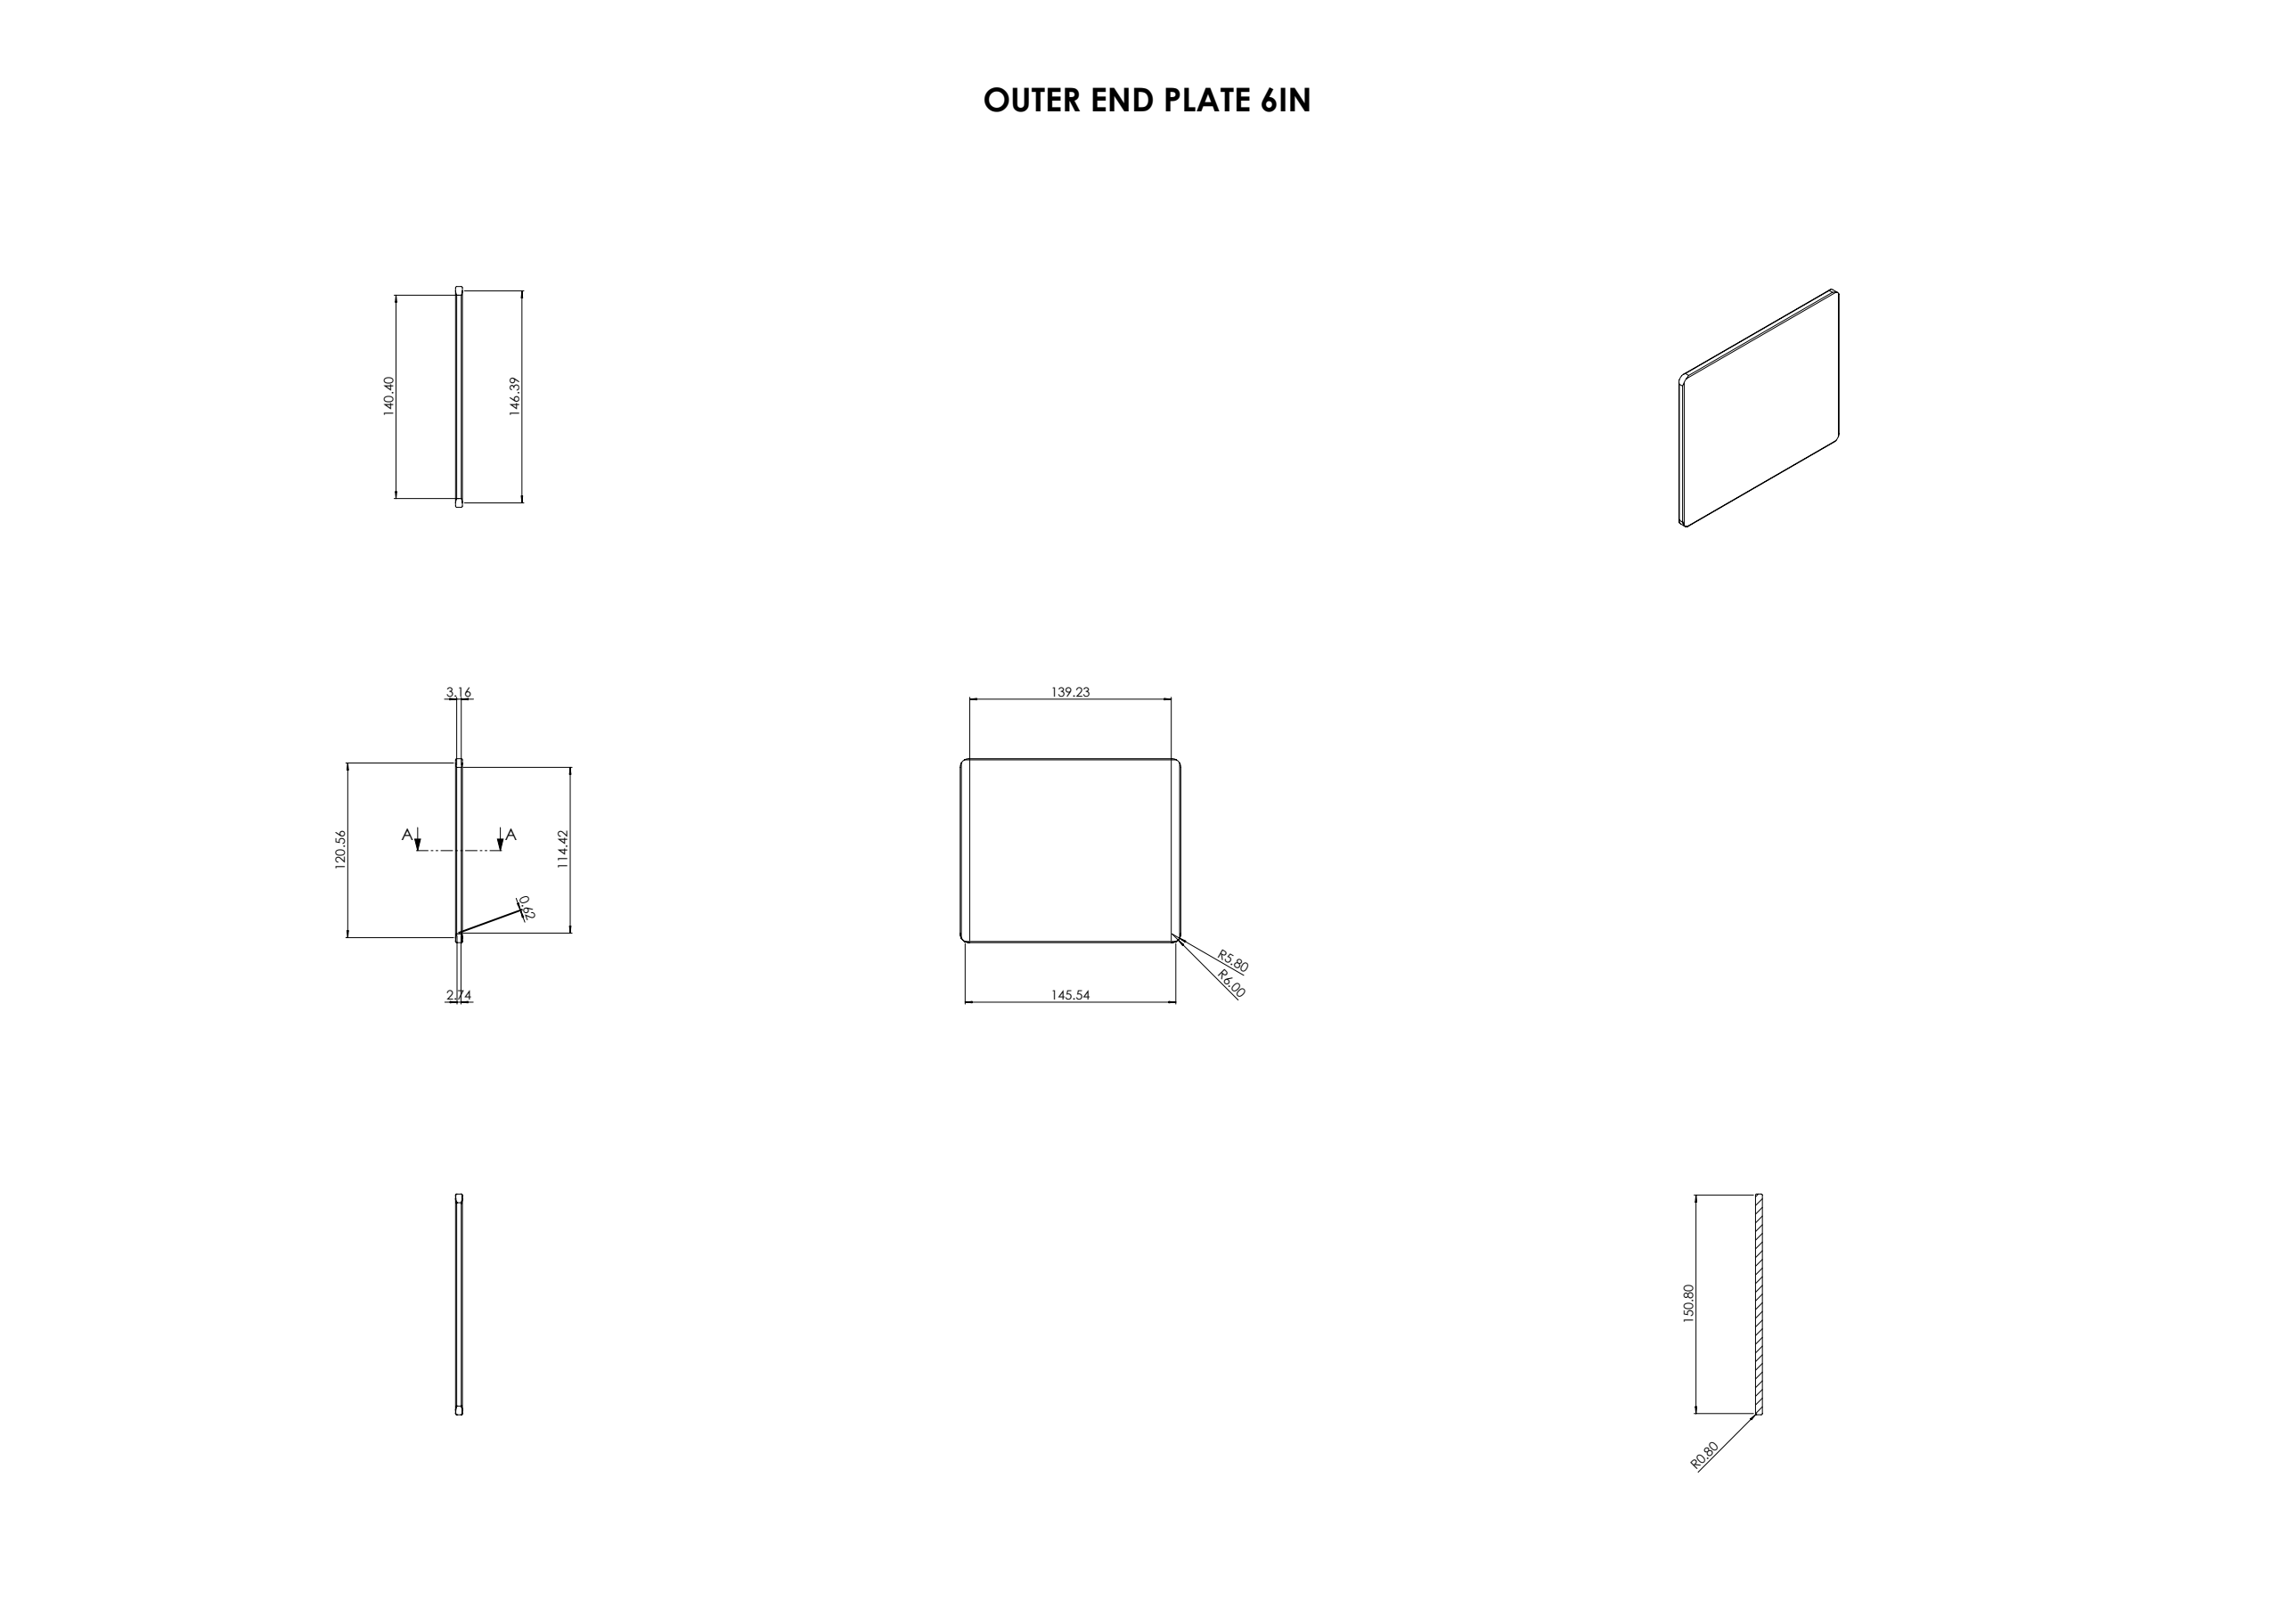
ISO-10303-21;
HEADER;
/* Generated by software containing ST-Developer
 * from STEP Tools, Inc. (www.steptools.com) 
 */

FILE_DESCRIPTION(
/* description */ (''),
/* implementation_level */ '2;1');

FILE_NAME(
/* name */ '02_Outer_End_Plate_6in.step',
/* time_stamp */ '2026-10-25T01:30:15-07:00',
/* author */ (''),
/* organization */ (''),
/* preprocessor_version */ 'ST-DEVELOPER v20.2',
/* originating_system */ 'Autodesk Translation Framework v15.15.0.0',
/* authorisation */ '');

FILE_SCHEMA (('AUTOMOTIVE_DESIGN { 1 0 10303 214 3 1 1 }'));
ENDSEC;

DATA;
#10=MECHANICAL_DESIGN_GEOMETRIC_PRESENTATION_REPRESENTATION('',(#564),#32309);
#88=B_SPLINE_CURVE_WITH_KNOTS('',3,(#18634,#18635,#18636,#18637,#18638,
#18639,#18640,#18641,#18642,#18643,#18644,#18645,#18646,#18647,#18648,#18649,
#18650,#18651,#18652,#18653,#18654,#18655,#18656,#18657,#18658,#18659,#18660,
#18661,#18662,#18663,#18664,#18665,#18666,#18667,#18668,#18669,#18670,#18671,
#18672,#18673,#18674,#18675,#18676,#18677,#18678,#18679,#18680,#18681,#18682,
#18683,#18684,#18685,#18686,#18687,#18688,#18689,#18690,#18691,#18692,#18693,
#18694,#18695,#18696,#18697,#18698,#18699,#18700,#18701,#18702,#18703,#18704,
#18705,#18706,#18707,#18708,#18709,#18710,#18711,#18712,#18713,#18714,#18715),
 .UNSPECIFIED.,.F.,.F.,(4,3,3,3,3,3,3,3,3,3,3,3,3,3,3,3,3,3,3,3,3,3,3,3,
3,3,3,4),(0.,0.0295705059520471,0.06051594873034,0.0926038163611335,0.126139587235275,
0.161619669140697,0.19997110729461,0.243460414926569,0.31097643988682,0.354040412393894,
0.394412886619275,0.429686040742309,0.462833625340497,0.494651029781358,
0.527129557828368,0.560643520110525,0.596019930687279,0.634095034705998,
0.676984118479283,0.757738088859462,0.799051739150417,0.836280907609681,
0.871099049046634,0.903485295335691,0.934889314251083,0.965468175632905,
0.995091329104342,1.),.UNSPECIFIED.);
#89=B_SPLINE_CURVE_WITH_KNOTS('',3,(#18717,#18718,#18719,#18720),
 .UNSPECIFIED.,.F.,.F.,(4,4),(-1.,0.),.UNSPECIFIED.);
#90=B_SPLINE_CURVE_WITH_KNOTS('',3,(#18722,#18723,#18724,#18725,#18726,
#18727,#18728,#18729,#18730,#18731,#18732,#18733,#18734,#18735,#18736,#18737,
#18738,#18739,#18740,#18741,#18742,#18743,#18744,#18745,#18746,#18747,#18748,
#18749,#18750,#18751,#18752,#18753,#18754,#18755,#18756,#18757,#18758,#18759,
#18760,#18761,#18762,#18763,#18764,#18765,#18766,#18767,#18768,#18769,#18770,
#18771,#18772,#18773),.UNSPECIFIED.,.F.,.F.,(4,3,3,3,3,3,3,3,3,3,3,3,3,
3,3,3,3,4),(0.,0.0499444618814776,0.102213228769125,0.161337745851018,0.226027786935006,
0.32277431356813,0.388018393772404,0.444871191794535,0.498045966144255,
0.551308035192963,0.608971249854249,0.676370629164652,0.757277971873489,
0.819640070739892,0.87628793152519,0.929442915859961,0.979183143018599,
1.),.UNSPECIFIED.);
#91=B_SPLINE_CURVE_WITH_KNOTS('',3,(#18813,#18814,#18815,#18816,#18817,
#18818,#18819,#18820,#18821,#18822,#18823,#18824,#18825,#18826,#18827,#18828,
#18829,#18830,#18831,#18832,#18833,#18834,#18835,#18836,#18837,#18838,#18839,
#18840,#18841,#18842,#18843,#18844,#18845,#18846,#18847,#18848,#18849,#18850,
#18851,#18852,#18853,#18854,#18855,#18856,#18857,#18858,#18859,#18860,#18861,
#18862,#18863,#18864),.UNSPECIFIED.,.F.,.F.,(4,3,3,3,3,3,3,3,3,3,3,3,3,
3,3,3,3,4),(0.,0.0499441833889704,0.102212663354794,0.161336814770105,0.226026300658832,
0.322773013076478,0.388016980146257,0.444869605985199,0.498043900535364,
0.551305760953485,0.608968431114082,0.676366602896629,0.757274952172472,
0.819637092644588,0.876284888158847,0.929439770312476,0.979179831895377,
1.),.UNSPECIFIED.);
#92=B_SPLINE_CURVE_WITH_KNOTS('',3,(#18866,#18867,#18868,#18869),
 .UNSPECIFIED.,.F.,.F.,(4,4),(0.,1.),.UNSPECIFIED.);
#93=B_SPLINE_CURVE_WITH_KNOTS('',3,(#18871,#18872,#18873,#18874,#18875,
#18876,#18877,#18878,#18879,#18880,#18881,#18882,#18883,#18884,#18885,#18886,
#18887,#18888,#18889,#18890,#18891,#18892,#18893,#18894,#18895,#18896,#18897,
#18898,#18899,#18900,#18901,#18902,#18903,#18904,#18905,#18906,#18907,#18908,
#18909,#18910,#18911,#18912,#18913,#18914,#18915,#18916,#18917,#18918,#18919,
#18920,#18921,#18922,#18923,#18924,#18925,#18926,#18927,#18928,#18929,#18930,
#18931,#18932,#18933,#18934,#18935,#18936,#18937,#18938,#18939,#18940,#18941,
#18942,#18943,#18944,#18945,#18946,#18947,#18948,#18949,#18950,#18951,#18952),
 .UNSPECIFIED.,.F.,.F.,(4,3,3,3,3,3,3,3,3,3,3,3,3,3,3,3,3,3,3,3,3,3,3,3,
3,3,3,4),(0.,0.0295773880527055,0.0605304168417959,0.0926266477934975,0.12617192252577,
0.16166335905183,0.200029751866471,0.243548698202303,0.31096188049889,0.354026762967709,
0.394400090282227,0.429679987033159,0.462839402284378,0.494661356434203,
0.527132671759088,0.560640873791091,0.596011156294116,0.634079510048534,
0.676959318035126,0.757719488526345,0.799022961860359,0.836244255344789,
0.871055470881663,0.903435211406727,0.934833076384915,0.965406058046024,
0.995023143022087,1.),.UNSPECIFIED.);
#94=B_SPLINE_CURVE_WITH_KNOTS('',3,(#18979,#18980,#18981,#18982,#18983,
#18984),.UNSPECIFIED.,.F.,.F.,(4,2,4),(9.99629094513137E-5,0.155241085196768,
0.273153287835105),.UNSPECIFIED.);
#95=B_SPLINE_CURVE_WITH_KNOTS('',3,(#18987,#18988,#18989,#18990,#18991,
#18992),.UNSPECIFIED.,.F.,.F.,(4,2,4),(-0.273153287835105,-0.155241085196768,
-9.99629094513137E-5),.UNSPECIFIED.);
#96=B_SPLINE_CURVE_WITH_KNOTS('',3,(#19018,#19019,#19020,#19021),
 .UNSPECIFIED.,.F.,.F.,(4,4),(-0.310482170393534,-0.273153287835093),
 .UNSPECIFIED.);
#97=B_SPLINE_CURVE_WITH_KNOTS('',3,(#19022,#19023,#19024,#19025),
 .UNSPECIFIED.,.F.,.F.,(4,4),(0.273153287835093,0.310482170393534),
 .UNSPECIFIED.);
#98=B_SPLINE_CURVE_WITH_KNOTS('',3,(#19051,#19052,#19053,#19054,#19055,
#19056),.UNSPECIFIED.,.F.,.F.,(4,2,4),(-0.954291288267864,-0.799150016166132,
-0.681237813527798),.UNSPECIFIED.);
#99=B_SPLINE_CURVE_WITH_KNOTS('',3,(#19059,#19060,#19061,#19062,#19063,
#19064),.UNSPECIFIED.,.F.,.F.,(4,2,4),(0.681237813527798,0.799150016166132,
0.954291288267864),.UNSPECIFIED.);
#100=B_SPLINE_CURVE_WITH_KNOTS('',3,(#19081,#19082,#19083,#19084),
 .UNSPECIFIED.,.F.,.F.,(4,4),(-0.681237813527811,-0.643908930969367),
 .UNSPECIFIED.);
#101=B_SPLINE_CURVE_WITH_KNOTS('',3,(#19085,#19086,#19087,#19088),
 .UNSPECIFIED.,.F.,.F.,(4,4),(0.643908930969367,0.681237813527811),
 .UNSPECIFIED.);
#102=B_SPLINE_CURVE_WITH_KNOTS('',3,(#19093,#19094,#19095,#19096,#19097,
#19098,#19099,#19100,#19101,#19102,#19103,#19104,#19105,#19106,#19107,#19108,
#19109,#19110,#19111,#19112,#19113,#19114,#19115,#19116,#19117,#19118,#19119,
#19120,#19121,#19122,#19123,#19124,#19125,#19126,#19127,#19128,#19129,#19130,
#19131,#19132,#19133,#19134,#19135,#19136,#19137,#19138,#19139,#19140,#19141,
#19142,#19143,#19144,#19145,#19146,#19147,#19148,#19149,#19150,#19151,#19152,
#19153,#19154,#19155,#19156,#19157,#19158,#19159,#19160,#19161,#19162,#19163,
#19164,#19165,#19166,#19167,#19168,#19169,#19170,#19171,#19172,#19173,#19174),
 .UNSPECIFIED.,.F.,.F.,(4,3,3,3,3,3,3,3,3,3,3,3,3,3,3,3,3,3,3,3,3,3,3,3,
3,3,3,4),(0.,0.0295773880962405,0.0605304169310475,0.0926266479315681,0.126171922717038,
0.161663359303526,0.200029752189728,0.243548698625291,0.310961878288235,
0.35402676089522,0.394400088339269,0.429679985266982,0.462839400402085,
0.494661354749945,0.527132670284999,0.560640872291038,0.596011154748267,
0.634079508418766,0.676959316170582,0.757719487127936,0.79902296069953,
0.836244254323238,0.871055469962877,0.903435210560169,0.9348330756024,0.965406057321837,
0.995023142345411,1.),.UNSPECIFIED.);
#103=B_SPLINE_CURVE_WITH_KNOTS('',3,(#19176,#19177,#19178,#19179,#19180,
#19181),.UNSPECIFIED.,.F.,.F.,(4,2,4),(-0.273153287835103,-0.155241085196768,
-9.99629094513097E-5),.UNSPECIFIED.);
#104=B_SPLINE_CURVE_WITH_KNOTS('',3,(#19199,#19200,#19201,#19202,#19203,
#19204,#19205,#19206,#19207,#19208,#19209,#19210,#19211,#19212,#19213,#19214,
#19215,#19216,#19217,#19218,#19219,#19220,#19221,#19222,#19223,#19224,#19225,
#19226,#19227,#19228,#19229,#19230,#19231,#19232,#19233,#19234,#19235,#19236,
#19237,#19238,#19239,#19240,#19241,#19242,#19243,#19244,#19245,#19246,#19247,
#19248,#19249,#19250),.UNSPECIFIED.,.F.,.F.,(4,3,3,3,3,3,3,3,3,3,3,3,3,
3,3,3,3,4),(0.,0.0499444622917576,0.102213229604467,0.161337747231124,0.226027789147348,
0.32277431550393,0.388018395851454,0.444871194115429,0.498045969164268,
0.551308038550752,0.608971254052268,0.676370635217512,0.757277976413134,
0.81964007522294,0.876287936115381,0.929442920613543,0.979183148031846,
1.),.UNSPECIFIED.);
#105=B_SPLINE_CURVE_WITH_KNOTS('',3,(#19252,#19253,#19254,#19255,#19256,
#19257),.UNSPECIFIED.,.F.,.F.,(4,2,4),(0.681229980645395,0.79914218328373,
0.954283455385462),.UNSPECIFIED.);
#106=B_SPLINE_CURVE_WITH_KNOTS('',3,(#19259,#19260,#19261,#19262),
 .UNSPECIFIED.,.F.,.F.,(4,4),(0.643901098086962,0.681229980645409),
 .UNSPECIFIED.);
#107=B_SPLINE_CURVE_WITH_KNOTS('',3,(#19266,#19267,#19268,#19269),
 .UNSPECIFIED.,.F.,.F.,(4,4),(0.269588855200382,0.305932679404608),
 .UNSPECIFIED.);
#108=B_SPLINE_CURVE_WITH_KNOTS('',3,(#19271,#19272,#19273,#19274,#19275,
#19276),.UNSPECIFIED.,.F.,.F.,(4,2,4),(9.97881403247492E-5,0.166940126137213,
0.269588855200419),.UNSPECIFIED.);
#109=B_SPLINE_CURVE_WITH_KNOTS('',3,(#19277,#19278,#19279,#19280,#19281,
#19282,#19283,#19284,#19285,#19286,#19287,#19288,#19289,#19290,#19291,#19292,
#19293,#19294,#19295,#19296,#19297,#19298,#19299,#19300,#19301,#19302,#19303,
#19304,#19305,#19306,#19307,#19308,#19309,#19310,#19311,#19312,#19313,#19314,
#19315,#19316,#19317,#19318,#19319,#19320,#19321,#19322,#19323,#19324,#19325,
#19326,#19327,#19328),.UNSPECIFIED.,.F.,.F.,(4,3,3,3,3,3,3,3,3,3,3,3,3,
3,3,3,3,4),(0.,0.0499444877726433,0.102213281220285,0.161337835137364,0.226027936148337,
0.322774444129795,0.38801851522186,0.444871319243691,0.498046130430203,
0.551308243614294,0.608971537556607,0.676371082027953,0.757278311520965,
0.819640416091138,0.876288295150041,0.92944330183216,0.979183558774527,
1.),.UNSPECIFIED.);
#110=B_SPLINE_CURVE_WITH_KNOTS('',3,(#19351,#19352,#19353,#19354,#19355,
#19356,#19357,#19358,#19359,#19360,#19361,#19362,#19363,#19364,#19365,#19366,
#19367,#19368,#19369,#19370,#19371,#19372,#19373,#19374,#19375,#19376,#19377,
#19378,#19379,#19380,#19381,#19382,#19383,#19384,#19385,#19386,#19387,#19388,
#19389,#19390,#19391,#19392,#19393,#19394,#19395,#19396,#19397,#19398,#19399,
#19400,#19401,#19402,#19403,#19404,#19405,#19406,#19407,#19408,#19409,#19410,
#19411,#19412,#19413,#19414,#19415,#19416,#19417,#19418,#19419,#19420,#19421,
#19422,#19423,#19424,#19425,#19426,#19427,#19428,#19429,#19430,#19431,#19432),
 .UNSPECIFIED.,.F.,.F.,(4,3,3,3,3,3,3,3,3,3,3,3,3,3,3,3,3,3,3,3,3,3,3,3,
3,3,3,4),(0.,0.0295705062457886,0.0605159494602176,0.0926038176850879,0.126139589401718,
0.161619672576972,0.199971112846056,0.243460425882021,0.310976395562794,
0.35404037084012,0.394412847662612,0.429686002557242,0.462833578893964,
0.494650986322964,0.527129524428408,0.560643490399518,0.596019903970715,
0.634095009431096,0.67698408832498,0.757738066243735,0.799051737694099,
0.836280920233922,0.87109907297074,0.903485328812536,0.934889356536429,
0.965468226164381,0.995091387717599,1.),.UNSPECIFIED.);
#111=B_SPLINE_CURVE_WITH_KNOTS('',3,(#19434,#19435,#19436,#19437),
 .UNSPECIFIED.,.F.,.F.,(4,4),(-1.,0.),.UNSPECIFIED.);
#112=B_SPLINE_CURVE_WITH_KNOTS('',3,(#19439,#19440,#19441,#19442,#19443,
#19444,#19445,#19446,#19447,#19448,#19449,#19450,#19451,#19452,#19453,#19454,
#19455,#19456,#19457,#19458,#19459,#19460,#19461,#19462,#19463,#19464,#19465,
#19466,#19467,#19468,#19469,#19470,#19471,#19472,#19473,#19474,#19475,#19476,
#19477,#19478,#19479,#19480,#19481,#19482,#19483,#19484,#19485,#19486,#19487,
#19488,#19489,#19490),.UNSPECIFIED.,.F.,.F.,(4,3,3,3,3,3,3,3,3,3,3,3,3,
3,3,3,3,4),(0.,0.049944493509105,0.102213293185184,0.161337852934914,0.226027959979003,
0.322774464981628,0.388018552338671,0.444871367106078,0.498046192643883,
0.551308282903018,0.608971555280469,0.676371064186631,0.757278298139973,
0.81964039022404,0.87628825630229,0.929443250152998,0.979183493767421,1.),
 .UNSPECIFIED.);
#113=B_SPLINE_CURVE_WITH_KNOTS('',3,(#19529,#19530,#19531,#19532,#19533,
#19534,#19535,#19536,#19537,#19538,#19539,#19540,#19541,#19542,#19543,#19544,
#19545,#19546,#19547,#19548,#19549,#19550,#19551,#19552,#19553,#19554,#19555,
#19556,#19557,#19558,#19559,#19560,#19561,#19562,#19563,#19564,#19565,#19566,
#19567,#19568,#19569,#19570,#19571,#19572,#19573,#19574,#19575,#19576,#19577,
#19578,#19579,#19580),.UNSPECIFIED.,.F.,.F.,(4,3,3,3,3,3,3,3,3,3,3,3,3,
3,3,3,3,4),(0.,0.0499441828918079,0.102212662342561,0.161336813097488,0.226026297979579,
0.322773010732132,0.388016977629376,0.444869603175185,0.498043896877559,
0.551305756885345,0.608968426026964,0.676366595561391,0.757274946671043,
0.819637087211295,0.876284882595595,0.929439764551152,0.979179825819233,
1.),.UNSPECIFIED.);
#114=B_SPLINE_CURVE_WITH_KNOTS('',3,(#19581,#19582,#19583,#19584),
 .UNSPECIFIED.,.F.,.F.,(4,4),(0.,1.),.UNSPECIFIED.);
#115=B_SPLINE_CURVE_WITH_KNOTS('',3,(#19610,#19611,#19612,#19613,#19614,
#19615),.UNSPECIFIED.,.F.,.F.,(4,2,4),(9.99629094513097E-5,0.155241085196768,
0.273153287835103),.UNSPECIFIED.);
#116=B_SPLINE_CURVE_WITH_KNOTS('',3,(#19642,#19643,#19644,#19645),
 .UNSPECIFIED.,.F.,.F.,(4,4),(-0.310482170393536,-0.273153287835089),
 .UNSPECIFIED.);
#117=B_SPLINE_CURVE_WITH_KNOTS('',3,(#19646,#19647,#19648,#19649),
 .UNSPECIFIED.,.F.,.F.,(4,4),(0.273153287835089,0.310482170393536),
 .UNSPECIFIED.);
#118=B_SPLINE_CURVE_WITH_KNOTS('',3,(#19675,#19676,#19677,#19678,#19679,
#19680),.UNSPECIFIED.,.F.,.F.,(4,2,4),(-0.945184496035906,-0.778344160365421,
-0.675695431302217),.UNSPECIFIED.);
#119=B_SPLINE_CURVE_WITH_KNOTS('',3,(#19683,#19684,#19685,#19686,#19687,
#19688),.UNSPECIFIED.,.F.,.F.,(4,2,4),(0.675695431302217,0.778344160365421,
0.945184496035906),.UNSPECIFIED.);
#120=B_SPLINE_CURVE_WITH_KNOTS('',3,(#19705,#19706,#19707,#19708),
 .UNSPECIFIED.,.F.,.F.,(4,4),(-0.675695431302254,-0.639351607098029),
 .UNSPECIFIED.);
#121=B_SPLINE_CURVE_WITH_KNOTS('',3,(#19709,#19710,#19711,#19712),
 .UNSPECIFIED.,.F.,.F.,(4,4),(0.639351607098029,0.675695431302254),
 .UNSPECIFIED.);
#122=B_SPLINE_CURVE_WITH_KNOTS('',3,(#19744,#19745,#19746,#19747,#19748,
#19749,#19750,#19751,#19752,#19753,#19754,#19755,#19756,#19757,#19758,#19759,
#19760,#19761,#19762,#19763,#19764,#19765,#19766,#19767,#19768,#19769,#19770,
#19771,#19772,#19773,#19774,#19775,#19776,#19777,#19778,#19779,#19780,#19781,
#19782,#19783,#19784,#19785,#19786,#19787,#19788,#19789,#19790,#19791,#19792,
#19793,#19794,#19795,#19796,#19797,#19798,#19799,#19800,#19801,#19802,#19803,
#19804,#19805,#19806,#19807,#19808,#19809,#19810,#19811,#19812,#19813,#19814,
#19815,#19816,#19817,#19818,#19819,#19820,#19821,#19822,#19823,#19824,#19825),
 .UNSPECIFIED.,.F.,.F.,(4,3,3,3,3,3,3,3,3,3,3,3,3,3,3,3,3,3,3,3,3,3,3,3,
3,3,3,4),(0.,0.0295705062009041,0.0605159493680217,0.0926038175409483,0.126139589200587,
0.161619672306982,0.199971112488613,0.243460425357206,0.310976394321422,
0.354040369676333,0.394412846571562,0.429686001479307,0.46283357764396,
0.49465098512599,0.527129523295935,0.560643489155532,0.596019902588203,
0.634095007862749,0.676984086399807,0.757738064799855,0.799051736386075,
0.836280918968163,0.871099071720543,0.903485327550832,0.934889355257872,
0.965468224868288,0.995091386390381,1.),.UNSPECIFIED.);
#123=B_SPLINE_CURVE_WITH_KNOTS('',3,(#19827,#19828,#19829,#19830),
 .UNSPECIFIED.,.F.,.F.,(4,4),(-1.,0.),.UNSPECIFIED.);
#124=B_SPLINE_CURVE_WITH_KNOTS('',3,(#19831,#19832,#19833,#19834,#19835,
#19836,#19837,#19838,#19839,#19840,#19841,#19842,#19843,#19844,#19845,#19846,
#19847,#19848,#19849,#19850,#19851,#19852,#19853,#19854,#19855,#19856,#19857,
#19858,#19859,#19860,#19861,#19862,#19863,#19864,#19865,#19866,#19867,#19868,
#19869,#19870,#19871,#19872,#19873,#19874,#19875,#19876,#19877,#19878,#19879,
#19880,#19881,#19882),.UNSPECIFIED.,.F.,.F.,(4,3,3,3,3,3,3,3,3,3,3,3,3,
3,3,3,3,4),(0.,0.0499444940857239,0.102213294358374,0.161337854873708,0.226027963088782,
0.322774467702684,0.388018555259764,0.444871370367514,0.498046196889068,
0.551308287624491,0.608971561184033,0.676371072696357,0.757278304522268,
0.819640396527144,0.87628826275593,0.92944325683678,0.979183500816116,1.),
 .UNSPECIFIED.);
#125=B_SPLINE_CURVE_WITH_KNOTS('',3,(#19921,#19922,#19923,#19924,#19925,
#19926,#19927,#19928,#19929,#19930,#19931,#19932,#19933,#19934,#19935,#19936,
#19937,#19938,#19939,#19940,#19941,#19942,#19943,#19944,#19945,#19946,#19947,
#19948,#19949,#19950,#19951,#19952,#19953,#19954,#19955,#19956,#19957,#19958,
#19959,#19960,#19961,#19962,#19963,#19964,#19965,#19966,#19967,#19968,#19969,
#19970,#19971,#19972),.UNSPECIFIED.,.F.,.F.,(4,3,3,3,3,3,3,3,3,3,3,3,3,
3,3,3,3,4),(0.,0.0499441826826897,0.102212661917196,0.161336812394391,0.22602629685116,
0.322773009744765,0.388016976569652,0.444869601991809,0.498043895337266,
0.551305755172809,0.608968423886568,0.676366592477159,0.757274944357869,
0.819637084926596,0.876284880256139,0.929439762127755,0.979179823263689,
1.),.UNSPECIFIED.);
#126=B_SPLINE_CURVE_WITH_KNOTS('',3,(#19974,#19975,#19976,#19977),
 .UNSPECIFIED.,.F.,.F.,(4,4),(0.,1.),.UNSPECIFIED.);
#127=B_SPLINE_CURVE_WITH_KNOTS('',3,(#19979,#19980,#19981,#19982,#19983,
#19984,#19985,#19986,#19987,#19988,#19989,#19990,#19991,#19992,#19993,#19994,
#19995,#19996,#19997,#19998,#19999,#20000,#20001,#20002,#20003,#20004,#20005,
#20006,#20007,#20008,#20009,#20010,#20011,#20012,#20013,#20014,#20015,#20016,
#20017,#20018,#20019,#20020,#20021,#20022,#20023,#20024,#20025,#20026,#20027,
#20028,#20029,#20030,#20031,#20032,#20033,#20034,#20035,#20036,#20037,#20038,
#20039,#20040,#20041,#20042,#20043,#20044,#20045,#20046,#20047,#20048,#20049,
#20050,#20051,#20052,#20053,#20054,#20055,#20056,#20057,#20058,#20059,#20060),
 .UNSPECIFIED.,.F.,.F.,(4,3,3,3,3,3,3,3,3,3,3,3,3,3,3,3,3,3,3,3,3,3,3,3,
3,3,3,4),(0.,0.0295773881143737,0.0605304169685423,0.0926266479893201,0.126171922797343,
0.161663359409954,0.200029752325282,0.243548698800364,0.310961877359763,
0.354026760024778,0.394400087523229,0.429679984526457,0.462839399613297,
0.494661354046568,0.527132669669348,0.560640871664874,0.596011154103228,
0.63407950774038,0.676959315395981,0.757719486546985,0.799022960216542,
0.836244253898911,0.871055469579005,0.90343521020651,0.934833075276548,
0.965406057021946,0.995023142066622,1.),.UNSPECIFIED.);
#128=B_SPLINE_CURVE_WITH_KNOTS('',3,(#20087,#20088,#20089,#20090,#20091,
#20092),.UNSPECIFIED.,.F.,.F.,(4,2,4),(9.99629094513175E-5,0.155241085196768,
0.273153287835103),.UNSPECIFIED.);
#129=B_SPLINE_CURVE_WITH_KNOTS('',3,(#20095,#20096,#20097,#20098,#20099,
#20100),.UNSPECIFIED.,.F.,.F.,(4,2,4),(-0.273153287835103,-0.155241085196768,
-9.99629094513175E-5),.UNSPECIFIED.);
#130=B_SPLINE_CURVE_WITH_KNOTS('',3,(#20126,#20127,#20128,#20129),
 .UNSPECIFIED.,.F.,.F.,(4,4),(-0.310482170393535,-0.273153287835089),
 .UNSPECIFIED.);
#131=B_SPLINE_CURVE_WITH_KNOTS('',3,(#20130,#20131,#20132,#20133),
 .UNSPECIFIED.,.F.,.F.,(4,4),(0.273153287835089,0.310482170393535),
 .UNSPECIFIED.);
#132=B_SPLINE_CURVE_WITH_KNOTS('',3,(#20159,#20160,#20161,#20162,#20163,
#20164),.UNSPECIFIED.,.F.,.F.,(4,2,4),(-0.945184496035905,-0.778344160365423,
-0.67569543130222),.UNSPECIFIED.);
#133=B_SPLINE_CURVE_WITH_KNOTS('',3,(#20167,#20168,#20169,#20170,#20171,
#20172),.UNSPECIFIED.,.F.,.F.,(4,2,4),(0.67569543130222,0.778344160365423,
0.945184496035905),.UNSPECIFIED.);
#134=B_SPLINE_CURVE_WITH_KNOTS('',3,(#20189,#20190,#20191,#20192),
 .UNSPECIFIED.,.F.,.F.,(4,4),(-0.675695431302257,-0.639351607098027),
 .UNSPECIFIED.);
#135=B_SPLINE_CURVE_WITH_KNOTS('',3,(#20193,#20194,#20195,#20196),
 .UNSPECIFIED.,.F.,.F.,(4,4),(0.639351607098027,0.675695431302257),
 .UNSPECIFIED.);
#136=B_SPLINE_CURVE_WITH_KNOTS('',3,(#20199,#20200,#20201,#20202,#20203,
#20204,#20205,#20206,#20207,#20208,#20209,#20210,#20211,#20212,#20213,#20214,
#20215,#20216,#20217,#20218,#20219,#20220,#20221,#20222,#20223,#20224,#20225,
#20226,#20227,#20228,#20229,#20230,#20231,#20232,#20233,#20234,#20235,#20236,
#20237,#20238,#20239,#20240,#20241,#20242,#20243,#20244,#20245,#20246,#20247,
#20248,#20249,#20250,#20251,#20252,#20253,#20254,#20255,#20256,#20257,#20258,
#20259,#20260,#20261,#20262,#20263,#20264,#20265,#20266,#20267,#20268,#20269,
#20270,#20271,#20272,#20273,#20274,#20275,#20276,#20277,#20278,#20279,#20280),
 .UNSPECIFIED.,.F.,.F.,(4,3,3,3,3,3,3,3,3,3,3,3,3,3,3,3,3,3,3,3,3,3,3,3,
3,3,3,4),(0.,0.0295774172384458,0.0605304778777659,0.0926267436200908,0.126172057442769,
0.161663540018093,0.200029992233166,0.243549050668545,0.310961698223174,
0.354026592084225,0.394399930078961,0.429679866520511,0.462839301683719,
0.494661290298148,0.527132633260964,0.560640855188699,0.596011159218635,
0.634079537198202,0.676959378678976,0.757719534009232,0.799023032825097,
0.836244348173232,0.871055583738876,0.90343534360451,0.934833227096761,
0.965406226610612,0.9950233300335,1.),.UNSPECIFIED.);
#137=B_SPLINE_CURVE_WITH_KNOTS('',3,(#20282,#20283,#20284,#20285,#20286,
#20287),.UNSPECIFIED.,.F.,.F.,(4,2,4),(-0.269588855200419,-0.166940126137213,
-9.97881403247492E-5),.UNSPECIFIED.);
#138=B_SPLINE_CURVE_WITH_KNOTS('',3,(#20313,#20314,#20315,#20316,#20317,
#20318,#20319,#20320,#20321,#20322,#20323,#20324,#20325,#20326,#20327,#20328,
#20329,#20330,#20331,#20332,#20333,#20334,#20335,#20336,#20337,#20338,#20339,
#20340,#20341,#20342,#20343,#20344,#20345,#20346,#20347,#20348,#20349,#20350,
#20351,#20352,#20353,#20354,#20355,#20356,#20357,#20358,#20359,#20360,#20361,
#20362,#20363,#20364,#20365,#20366,#20367,#20368,#20369,#20370,#20371,#20372,
#20373,#20374,#20375,#20376,#20377,#20378,#20379,#20380,#20381,#20382,#20383,
#20384,#20385,#20386,#20387,#20388,#20389,#20390,#20391,#20392,#20393,#20394),
 .UNSPECIFIED.,.F.,.F.,(4,3,3,3,3,3,3,3,3,3,3,3,3,3,3,3,3,3,3,3,3,3,3,3,
3,3,3,4),(0.,0.0295705059225161,0.060515948666961,0.0926038162606335,0.126139587093134,
0.161619668950802,0.199971107042965,0.243460414554639,0.310976439007705,
0.354040411569723,0.394412885846616,0.429686039982354,0.462833624458519,
0.494651028937031,0.527129557030648,0.560643519234301,0.596019929713648,
0.634095033602234,0.676984117122705,0.757738087842029,0.799051738229506,
0.836280906721543,0.871099048168231,0.903485294448113,0.934889313350476,
0.96546817471544,0.995091328163233,1.),.UNSPECIFIED.);
#139=B_SPLINE_CURVE_WITH_KNOTS('',3,(#20395,#20396,#20397,#20398),
 .UNSPECIFIED.,.F.,.F.,(4,4),(-1.,0.),.UNSPECIFIED.);
#140=B_SPLINE_CURVE_WITH_KNOTS('',3,(#20436,#20437,#20438,#20439),
 .UNSPECIFIED.,.F.,.F.,(4,4),(0.,1.),.UNSPECIFIED.);
#141=B_SPLINE_CURVE_WITH_KNOTS('',3,(#20487,#20488,#20489,#20490),
 .UNSPECIFIED.,.F.,.F.,(4,4),(-0.305932679404608,-0.269588855200382),
 .UNSPECIFIED.);
#142=B_SPLINE_CURVE_WITH_KNOTS('',3,(#20516,#20517,#20518,#20519,#20520,
#20521),.UNSPECIFIED.,.F.,.F.,(4,2,4),(-0.954283455385462,-0.79914218328373,
-0.681229980645395),.UNSPECIFIED.);
#143=B_SPLINE_CURVE_WITH_KNOTS('',3,(#20539,#20540,#20541,#20542),
 .UNSPECIFIED.,.F.,.F.,(4,4),(-0.681229980645409,-0.643901098086962),
 .UNSPECIFIED.);
#144=B_SPLINE_CURVE_WITH_KNOTS('',3,(#20556,#20557,#20558,#20559,#20560,
#20561),.UNSPECIFIED.,.F.,.F.,(4,2,4),(0.,0.155241085196768,0.310482170393537),
 .UNSPECIFIED.);
#145=B_SPLINE_CURVE_WITH_KNOTS('',3,(#20565,#20566,#20567,#20568,#20569,
#20570),.UNSPECIFIED.,.F.,.F.,(4,2,4),(0.643901098086962,0.79914218328373,
0.954383268480499),.UNSPECIFIED.);
#146=B_SPLINE_CURVE_WITH_KNOTS('',3,(#20572,#20573,#20574,#20575,#20576,
#20577),.UNSPECIFIED.,.F.,.F.,(4,2,4),(0.,0.15524108519677,0.31048217039354),
 .UNSPECIFIED.);
#147=B_SPLINE_CURVE_WITH_KNOTS('',3,(#20580,#20581,#20582,#20583,#20584,
#20585),.UNSPECIFIED.,.F.,.F.,(4,2,4),(0.643901098086964,0.799142183283734,
0.954383268480504),.UNSPECIFIED.);
#148=B_SPLINE_CURVE_WITH_KNOTS('',3,(#20591,#20592,#20593,#20594,#20595,
#20596),.UNSPECIFIED.,.F.,.F.,(4,2,4),(0.,0.155241085196768,0.310482170393535),
 .UNSPECIFIED.);
#149=B_SPLINE_CURVE_WITH_KNOTS('',3,(#20601,#20602,#20603,#20604,#20605,
#20606),.UNSPECIFIED.,.F.,.F.,(4,2,4),(0.643901098086961,0.799142183283728,
0.954383268480496),.UNSPECIFIED.);
#150=B_SPLINE_CURVE_WITH_KNOTS('',3,(#20608,#20609,#20610,#20611,#20612,
#20613),.UNSPECIFIED.,.F.,.F.,(4,2,4),(0.,0.166940126137215,0.305932679404607),
 .UNSPECIFIED.);
#151=B_SPLINE_CURVE_WITH_KNOTS('',3,(#20616,#20617,#20618,#20619,#20620,
#20621),.UNSPECIFIED.,.F.,.F.,(4,2,4),(0.643908930969365,0.799150016166133,
0.954391101362901),.UNSPECIFIED.);
#407=B_SPLINE_SURFACE_WITH_KNOTS('',3,3,((#18612,#18613,#18614,#18615,#18616),
(#18617,#18618,#18619,#18620,#18621),(#18622,#18623,#18624,#18625,#18626),
(#18627,#18628,#18629,#18630,#18631)),.UNSPECIFIED.,.F.,.F.,.F.,(4,4),(4,
1,4),(0.,1.),(0.,0.571428571428571,1.),.UNSPECIFIED.);
#408=B_SPLINE_SURFACE_WITH_KNOTS('',3,3,((#18775,#18776,#18777,#18778,#18779,
#18780,#18781,#18782,#18783),(#18784,#18785,#18786,#18787,#18788,#18789,
#18790,#18791,#18792),(#18793,#18794,#18795,#18796,#18797,#18798,#18799,
#18800,#18801),(#18802,#18803,#18804,#18805,#18806,#18807,#18808,#18809,
#18810)),.UNSPECIFIED.,.F.,.F.,.F.,(4,4),(4,1,1,1,1,1,4),(0.,1.),(0.,0.214285714285714,
0.357142857142857,0.571428571428571,0.785714285714286,0.857142857142857,
1.),.UNSPECIFIED.);
#409=B_SPLINE_SURFACE_WITH_KNOTS('',3,3,((#18954,#18955,#18956,#18957,#18958,
#18959),(#18960,#18961,#18962,#18963,#18964,#18965),(#18966,#18967,#18968,
#18969,#18970,#18971),(#18972,#18973,#18974,#18975,#18976,#18977)),
 .UNSPECIFIED.,.F.,.F.,.F.,(4,4),(4,2,4),(0.,1.),(9.99629094513137E-5,0.155241085196768,
0.273153287835105),.UNSPECIFIED.);
#410=B_SPLINE_SURFACE_WITH_KNOTS('',3,3,((#19002,#19003,#19004,#19005),
(#19006,#19007,#19008,#19009),(#19010,#19011,#19012,#19013),(#19014,#19015,
#19016,#19017)),.UNSPECIFIED.,.F.,.F.,.F.,(4,4),(4,4),(0.,1.),(0.273153287835093,
0.310482170393534),.UNSPECIFIED.);
#411=B_SPLINE_SURFACE_WITH_KNOTS('',3,3,((#19026,#19027,#19028,#19029,#19030,
#19031),(#19032,#19033,#19034,#19035,#19036,#19037),(#19038,#19039,#19040,
#19041,#19042,#19043),(#19044,#19045,#19046,#19047,#19048,#19049)),
 .UNSPECIFIED.,.F.,.F.,.F.,(4,4),(4,2,4),(0.,1.),(0.681237813527798,0.799150016166132,
0.954291288267864),.UNSPECIFIED.);
#412=B_SPLINE_SURFACE_WITH_KNOTS('',3,3,((#19065,#19066,#19067,#19068),
(#19069,#19070,#19071,#19072),(#19073,#19074,#19075,#19076),(#19077,#19078,
#19079,#19080)),.UNSPECIFIED.,.F.,.F.,.F.,(4,4),(4,4),(0.,1.),(0.643908930969367,
0.681237813527811),.UNSPECIFIED.);
#413=B_SPLINE_SURFACE_WITH_KNOTS('',3,3,((#19329,#19330,#19331,#19332,#19333),
(#19334,#19335,#19336,#19337,#19338),(#19339,#19340,#19341,#19342,#19343),
(#19344,#19345,#19346,#19347,#19348)),.UNSPECIFIED.,.F.,.F.,.F.,(4,4),(4,
1,4),(0.,1.),(0.,0.571428571428571,1.),.UNSPECIFIED.);
#414=B_SPLINE_SURFACE_WITH_KNOTS('',3,3,((#19492,#19493,#19494,#19495,#19496,
#19497,#19498,#19499,#19500),(#19501,#19502,#19503,#19504,#19505,#19506,
#19507,#19508,#19509),(#19510,#19511,#19512,#19513,#19514,#19515,#19516,
#19517,#19518),(#19519,#19520,#19521,#19522,#19523,#19524,#19525,#19526,
#19527)),.UNSPECIFIED.,.F.,.F.,.F.,(4,4),(4,1,1,1,1,1,4),(0.,1.),(0.,0.214285714285714,
0.357142857142857,0.571428571428571,0.785714285714286,0.857142857142857,
1.),.UNSPECIFIED.);
#415=B_SPLINE_SURFACE_WITH_KNOTS('',3,3,((#19585,#19586,#19587,#19588,#19589,
#19590),(#19591,#19592,#19593,#19594,#19595,#19596),(#19597,#19598,#19599,
#19600,#19601,#19602),(#19603,#19604,#19605,#19606,#19607,#19608)),
 .UNSPECIFIED.,.F.,.F.,.F.,(4,4),(4,2,4),(0.,1.),(9.99629094513097E-5,0.155241085196768,
0.273153287835103),.UNSPECIFIED.);
#416=B_SPLINE_SURFACE_WITH_KNOTS('',3,3,((#19626,#19627,#19628,#19629),
(#19630,#19631,#19632,#19633),(#19634,#19635,#19636,#19637),(#19638,#19639,
#19640,#19641)),.UNSPECIFIED.,.F.,.F.,.F.,(4,4),(4,4),(0.,1.),(0.273153287835089,
0.310482170393536),.UNSPECIFIED.);
#417=B_SPLINE_SURFACE_WITH_KNOTS('',3,3,((#19650,#19651,#19652,#19653,#19654,
#19655),(#19656,#19657,#19658,#19659,#19660,#19661),(#19662,#19663,#19664,
#19665,#19666,#19667),(#19668,#19669,#19670,#19671,#19672,#19673)),
 .UNSPECIFIED.,.F.,.F.,.F.,(4,4),(4,2,4),(0.,1.),(0.675695431302217,0.778344160365421,
0.945184496035906),.UNSPECIFIED.);
#418=B_SPLINE_SURFACE_WITH_KNOTS('',3,3,((#19689,#19690,#19691,#19692),
(#19693,#19694,#19695,#19696),(#19697,#19698,#19699,#19700),(#19701,#19702,
#19703,#19704)),.UNSPECIFIED.,.F.,.F.,.F.,(4,4),(4,4),(0.,1.),(0.639351607098029,
0.675695431302254),.UNSPECIFIED.);
#419=B_SPLINE_SURFACE_WITH_KNOTS('',3,3,((#19723,#19724,#19725,#19726,#19727),
(#19728,#19729,#19730,#19731,#19732),(#19733,#19734,#19735,#19736,#19737),
(#19738,#19739,#19740,#19741,#19742)),.UNSPECIFIED.,.F.,.F.,.F.,(4,4),(4,
1,4),(0.,1.),(0.,0.571428571428571,1.),.UNSPECIFIED.);
#420=B_SPLINE_SURFACE_WITH_KNOTS('',3,3,((#19883,#19884,#19885,#19886,#19887,
#19888,#19889,#19890,#19891),(#19892,#19893,#19894,#19895,#19896,#19897,
#19898,#19899,#19900),(#19901,#19902,#19903,#19904,#19905,#19906,#19907,
#19908,#19909),(#19910,#19911,#19912,#19913,#19914,#19915,#19916,#19917,
#19918)),.UNSPECIFIED.,.F.,.F.,.F.,(4,4),(4,1,1,1,1,1,4),(0.,1.),(0.,0.214285714285714,
0.357142857142857,0.571428571428571,0.785714285714286,0.857142857142857,
1.),.UNSPECIFIED.);
#421=B_SPLINE_SURFACE_WITH_KNOTS('',3,3,((#20062,#20063,#20064,#20065,#20066,
#20067),(#20068,#20069,#20070,#20071,#20072,#20073),(#20074,#20075,#20076,
#20077,#20078,#20079),(#20080,#20081,#20082,#20083,#20084,#20085)),
 .UNSPECIFIED.,.F.,.F.,.F.,(4,4),(4,2,4),(0.,1.),(9.99629094513175E-5,0.155241085196768,
0.273153287835103),.UNSPECIFIED.);
#422=B_SPLINE_SURFACE_WITH_KNOTS('',3,3,((#20110,#20111,#20112,#20113),
(#20114,#20115,#20116,#20117),(#20118,#20119,#20120,#20121),(#20122,#20123,
#20124,#20125)),.UNSPECIFIED.,.F.,.F.,.F.,(4,4),(4,4),(0.,1.),(0.273153287835089,
0.310482170393535),.UNSPECIFIED.);
#423=B_SPLINE_SURFACE_WITH_KNOTS('',3,3,((#20134,#20135,#20136,#20137,#20138,
#20139),(#20140,#20141,#20142,#20143,#20144,#20145),(#20146,#20147,#20148,
#20149,#20150,#20151),(#20152,#20153,#20154,#20155,#20156,#20157)),
 .UNSPECIFIED.,.F.,.F.,.F.,(4,4),(4,2,4),(0.,1.),(0.67569543130222,0.778344160365423,
0.945184496035905),.UNSPECIFIED.);
#424=B_SPLINE_SURFACE_WITH_KNOTS('',3,3,((#20173,#20174,#20175,#20176),
(#20177,#20178,#20179,#20180),(#20181,#20182,#20183,#20184),(#20185,#20186,
#20187,#20188)),.UNSPECIFIED.,.F.,.F.,.F.,(4,4),(4,4),(0.,1.),(0.639351607098027,
0.675695431302257),.UNSPECIFIED.);
#425=B_SPLINE_SURFACE_WITH_KNOTS('',3,3,((#20291,#20292,#20293,#20294,#20295),
(#20296,#20297,#20298,#20299,#20300),(#20301,#20302,#20303,#20304,#20305),
(#20306,#20307,#20308,#20309,#20310)),.UNSPECIFIED.,.F.,.F.,.F.,(4,4),(4,
1,4),(0.,1.),(0.,0.571428571428571,1.),.UNSPECIFIED.);
#426=B_SPLINE_SURFACE_WITH_KNOTS('',3,3,((#20400,#20401,#20402,#20403,#20404,
#20405,#20406,#20407,#20408),(#20409,#20410,#20411,#20412,#20413,#20414,
#20415,#20416,#20417),(#20418,#20419,#20420,#20421,#20422,#20423,#20424,
#20425,#20426),(#20427,#20428,#20429,#20430,#20431,#20432,#20433,#20434,
#20435)),.UNSPECIFIED.,.F.,.F.,.F.,(4,4),(4,1,1,1,1,1,4),(0.,1.),(0.,0.214285714285714,
0.357142857142857,0.571428571428571,0.785714285714286,0.857142857142857,
1.),.UNSPECIFIED.);
#427=B_SPLINE_SURFACE_WITH_KNOTS('',3,3,((#20440,#20441,#20442,#20443,#20444,
#20445),(#20446,#20447,#20448,#20449,#20450,#20451),(#20452,#20453,#20454,
#20455,#20456,#20457),(#20458,#20459,#20460,#20461,#20462,#20463)),
 .UNSPECIFIED.,.F.,.F.,.F.,(4,4),(4,2,4),(0.,1.),(9.97881403247492E-5,0.166940126137213,
0.269588855200419),.UNSPECIFIED.);
#428=B_SPLINE_SURFACE_WITH_KNOTS('',3,3,((#20471,#20472,#20473,#20474),
(#20475,#20476,#20477,#20478),(#20479,#20480,#20481,#20482),(#20483,#20484,
#20485,#20486)),.UNSPECIFIED.,.F.,.F.,.F.,(4,4),(4,4),(0.,1.),(0.269588855200382,
0.305932679404608),.UNSPECIFIED.);
#429=B_SPLINE_SURFACE_WITH_KNOTS('',3,3,((#20491,#20492,#20493,#20494,#20495,
#20496),(#20497,#20498,#20499,#20500,#20501,#20502),(#20503,#20504,#20505,
#20506,#20507,#20508),(#20509,#20510,#20511,#20512,#20513,#20514)),
 .UNSPECIFIED.,.F.,.F.,.F.,(4,4),(4,2,4),(0.,1.),(0.681229980645395,0.79914218328373,
0.954283455385462),.UNSPECIFIED.);
#430=B_SPLINE_SURFACE_WITH_KNOTS('',3,3,((#20523,#20524,#20525,#20526),
(#20527,#20528,#20529,#20530),(#20531,#20532,#20533,#20534),(#20535,#20536,
#20537,#20538)),.UNSPECIFIED.,.F.,.F.,.F.,(4,4),(4,4),(0.,1.),(0.643901098086962,
0.681229980645409),.UNSPECIFIED.);
#536=SHAPE_REPRESENTATION_RELATIONSHIP('SRR','None',#32363,#550);
#550=ADVANCED_BREP_SHAPE_REPRESENTATION('',(#578),#32296);
#564=STYLED_ITEM('',(#32516),#578);
#578=MANIFOLD_SOLID_BREP('Body1',#13805);
#656=CYLINDRICAL_SURFACE('',#14064,0.8);
#657=CYLINDRICAL_SURFACE('',#14066,6.00000000000001);
#658=CYLINDRICAL_SURFACE('',#14077,0.8);
#659=CYLINDRICAL_SURFACE('',#14078,6.00000000000001);
#660=CYLINDRICAL_SURFACE('',#14084,0.8);
#661=CYLINDRICAL_SURFACE('',#14085,6.);
#662=CYLINDRICAL_SURFACE('',#14087,0.8);
#663=CYLINDRICAL_SURFACE('',#14088,0.8);
#664=CYLINDRICAL_SURFACE('',#14089,5.99999999999998);
#665=CYLINDRICAL_SURFACE('',#14091,0.8);
#666=CYLINDRICAL_SURFACE('',#14092,0.8);
#667=CYLINDRICAL_SURFACE('',#14094,0.8);
#807=CIRCLE('',#14062,6.00000000000001);
#808=CIRCLE('',#14063,5.80000000000001);
#809=CIRCLE('',#14067,6.00000000000001);
#810=CIRCLE('',#14069,6.00000000000001);
#811=CIRCLE('',#14070,5.80000000000001);
#812=CIRCLE('',#14072,5.99999999999998);
#813=CIRCLE('',#14073,6.);
#814=CIRCLE('',#14075,5.80000000000001);
#815=CIRCLE('',#14076,6.00000000000001);
#816=CIRCLE('',#14080,5.80000000000001);
#817=CIRCLE('',#14082,6.);
#818=CIRCLE('',#14083,5.99999999999998);
#1113=CONICAL_SURFACE('',#14061,5.90000000000001,0.785398163397448);
#1114=CONICAL_SURFACE('',#14068,5.90000000000001,0.785398163397451);
#1115=CONICAL_SURFACE('',#14074,5.90000000000001,0.785398163397451);
#1116=CONICAL_SURFACE('',#14079,5.90000000000001,0.785398163397448);
#1293=FACE_OUTER_BOUND('',#2096,.T.);
#1294=FACE_OUTER_BOUND('',#2097,.T.);
#1295=FACE_OUTER_BOUND('',#2098,.T.);
#1296=FACE_OUTER_BOUND('',#2099,.T.);
#1297=FACE_OUTER_BOUND('',#2100,.T.);
#1298=FACE_OUTER_BOUND('',#2101,.T.);
#1299=FACE_OUTER_BOUND('',#2102,.T.);
#1300=FACE_OUTER_BOUND('',#2103,.T.);
#1301=FACE_OUTER_BOUND('',#2104,.T.);
#1302=FACE_OUTER_BOUND('',#2105,.T.);
#1303=FACE_OUTER_BOUND('',#2106,.T.);
#1304=FACE_OUTER_BOUND('',#2107,.T.);
#1305=FACE_OUTER_BOUND('',#2108,.T.);
#1306=FACE_OUTER_BOUND('',#2109,.T.);
#1307=FACE_OUTER_BOUND('',#2110,.T.);
#1308=FACE_OUTER_BOUND('',#2111,.T.);
#1309=FACE_OUTER_BOUND('',#2112,.T.);
#1310=FACE_OUTER_BOUND('',#2113,.T.);
#1311=FACE_OUTER_BOUND('',#2114,.T.);
#1312=FACE_OUTER_BOUND('',#2115,.T.);
#1313=FACE_OUTER_BOUND('',#2116,.T.);
#1314=FACE_OUTER_BOUND('',#2117,.T.);
#1315=FACE_OUTER_BOUND('',#2118,.T.);
#1316=FACE_OUTER_BOUND('',#2119,.T.);
#1317=FACE_OUTER_BOUND('',#2120,.T.);
#1318=FACE_OUTER_BOUND('',#2121,.T.);
#1319=FACE_OUTER_BOUND('',#2122,.T.);
#1320=FACE_OUTER_BOUND('',#2123,.T.);
#1321=FACE_OUTER_BOUND('',#2124,.T.);
#1322=FACE_OUTER_BOUND('',#2125,.T.);
#1323=FACE_OUTER_BOUND('',#2126,.T.);
#1324=FACE_OUTER_BOUND('',#2127,.T.);
#1325=FACE_OUTER_BOUND('',#2128,.T.);
#1326=FACE_OUTER_BOUND('',#2129,.T.);
#1327=FACE_OUTER_BOUND('',#2130,.T.);
#1328=FACE_OUTER_BOUND('',#2131,.T.);
#1329=FACE_OUTER_BOUND('',#2132,.T.);
#1330=FACE_OUTER_BOUND('',#2133,.T.);
#1331=FACE_OUTER_BOUND('',#2134,.T.);
#1332=FACE_OUTER_BOUND('',#2135,.T.);
#1333=FACE_OUTER_BOUND('',#2136,.T.);
#1334=FACE_OUTER_BOUND('',#2137,.T.);
#1335=FACE_OUTER_BOUND('',#2138,.T.);
#1336=FACE_OUTER_BOUND('',#2139,.T.);
#1337=FACE_OUTER_BOUND('',#2140,.T.);
#1338=FACE_OUTER_BOUND('',#2141,.T.);
#2096=EDGE_LOOP('',(#8909,#8910,#8911,#8912));
#2097=EDGE_LOOP('',(#8913,#8914,#8915,#8916));
#2098=EDGE_LOOP('',(#8917,#8918,#8919,#8920));
#2099=EDGE_LOOP('',(#8921,#8922,#8923,#8924));
#2100=EDGE_LOOP('',(#8925,#8926,#8927,#8928));
#2101=EDGE_LOOP('',(#8929,#8930,#8931,#8932));
#2102=EDGE_LOOP('',(#8933,#8934,#8935,#8936));
#2103=EDGE_LOOP('',(#8937,#8938,#8939,#8940,#8941,#8942));
#2104=EDGE_LOOP('',(#8943,#8944,#8945,#8946,#8947,#8948,#8949,#8950));
#2105=EDGE_LOOP('',(#8951,#8952,#8953,#8954,#8955,#8956,#8957,#8958,#8959,
#8960,#8961,#8962,#8963,#8964,#8965,#8966));
#2106=EDGE_LOOP('',(#8967,#8968,#8969,#8970));
#2107=EDGE_LOOP('',(#8971,#8972,#8973,#8974));
#2108=EDGE_LOOP('',(#8975,#8976,#8977,#8978));
#2109=EDGE_LOOP('',(#8979,#8980,#8981,#8982));
#2110=EDGE_LOOP('',(#8983,#8984,#8985,#8986));
#2111=EDGE_LOOP('',(#8987,#8988,#8989,#8990));
#2112=EDGE_LOOP('',(#8991,#8992,#8993,#8994));
#2113=EDGE_LOOP('',(#8995,#8996,#8997,#8998,#8999,#9000,#9001,#9002,#9003,
#9004,#9005,#9006));
#2114=EDGE_LOOP('',(#9007,#9008,#9009,#9010));
#2115=EDGE_LOOP('',(#9011,#9012,#9013,#9014));
#2116=EDGE_LOOP('',(#9015,#9016,#9017,#9018));
#2117=EDGE_LOOP('',(#9019,#9020,#9021,#9022));
#2118=EDGE_LOOP('',(#9023,#9024,#9025,#9026));
#2119=EDGE_LOOP('',(#9027,#9028,#9029,#9030));
#2120=EDGE_LOOP('',(#9031,#9032,#9033,#9034));
#2121=EDGE_LOOP('',(#9035,#9036,#9037,#9038,#9039,#9040));
#2122=EDGE_LOOP('',(#9041,#9042,#9043,#9044,#9045,#9046,#9047,#9048,#9049,
#9050,#9051,#9052,#9053,#9054,#9055,#9056));
#2123=EDGE_LOOP('',(#9057,#9058,#9059,#9060));
#2124=EDGE_LOOP('',(#9061,#9062,#9063,#9064));
#2125=EDGE_LOOP('',(#9065,#9066,#9067,#9068));
#2126=EDGE_LOOP('',(#9069,#9070,#9071,#9072));
#2127=EDGE_LOOP('',(#9073,#9074,#9075,#9076));
#2128=EDGE_LOOP('',(#9077,#9078,#9079,#9080));
#2129=EDGE_LOOP('',(#9081,#9082,#9083,#9084));
#2130=EDGE_LOOP('',(#9085,#9086,#9087,#9088,#9089,#9090,#9091,#9092,#9093,
#9094,#9095,#9096));
#2131=EDGE_LOOP('',(#9097,#9098,#9099,#9100,#9101));
#2132=EDGE_LOOP('',(#9102,#9103,#9104,#9105,#9106,#9107,#9108,#9109));
#2133=EDGE_LOOP('',(#9110,#9111,#9112,#9113,#9114,#9115));
#2134=EDGE_LOOP('',(#9116,#9117,#9118,#9119,#9120));
#2135=EDGE_LOOP('',(#9121,#9122,#9123,#9124));
#2136=EDGE_LOOP('',(#9125,#9126,#9127,#9128,#9129,#9130,#9131,#9132));
#2137=EDGE_LOOP('',(#9133,#9134,#9135,#9136));
#2138=EDGE_LOOP('',(#9137,#9138,#9139,#9140));
#2139=EDGE_LOOP('',(#9141,#9142,#9143,#9144,#9145));
#2140=EDGE_LOOP('',(#9146,#9147,#9148,#9149,#9150,#9151));
#2141=EDGE_LOOP('',(#9152,#9153,#9154,#9155,#9156));
#2977=LINE('',#18774,#4288);
#2978=LINE('',#18953,#4289);
#2979=LINE('',#18986,#4290);
#2980=LINE('',#18996,#4291);
#2981=LINE('',#19000,#4292);
#2982=LINE('',#19058,#4293);
#2983=LINE('',#19091,#4294);
#2984=LINE('',#19182,#4295);
#2985=LINE('',#19185,#4296);
#2986=LINE('',#19187,#4297);
#2987=LINE('',#19189,#4298);
#2988=LINE('',#19191,#4299);
#2989=LINE('',#19193,#4300);
#2990=LINE('',#19194,#4301);
#2991=LINE('',#19197,#4302);
#2992=LINE('',#19491,#4303);
#2993=LINE('',#19616,#4304);
#2994=LINE('',#19620,#4305);
#2995=LINE('',#19624,#4306);
#2996=LINE('',#19682,#4307);
#2997=LINE('',#19715,#4308);
#2998=LINE('',#19719,#4309);
#2999=LINE('',#19722,#4310);
#3000=LINE('',#20061,#4311);
#3001=LINE('',#20094,#4312);
#3002=LINE('',#20104,#4313);
#3003=LINE('',#20108,#4314);
#3004=LINE('',#20166,#4315);
#3005=LINE('',#20288,#4316);
#3006=LINE('',#20290,#4317);
#3007=LINE('',#20399,#4318);
#3008=LINE('',#20464,#4319);
#3009=LINE('',#20467,#4320);
#3010=LINE('',#20470,#4321);
#3011=LINE('',#20522,#4322);
#3012=LINE('',#20545,#4323);
#3013=LINE('',#20549,#4324);
#3014=LINE('',#20552,#4325);
#3015=LINE('',#20555,#4326);
#3016=LINE('',#20564,#4327);
#3017=LINE('',#20579,#4328);
#3018=LINE('',#20587,#4329);
#3019=LINE('',#20597,#4330);
#3020=LINE('',#20600,#4331);
#3021=LINE('',#20615,#4332);
#3022=LINE('',#20623,#4333);
#3023=LINE('',#20626,#4334);
#3024=LINE('',#20628,#4335);
#4288=VECTOR('',#15261,10.);
#4289=VECTOR('',#15262,10.);
#4290=VECTOR('',#15263,10.);
#4291=VECTOR('',#15266,10.);
#4292=VECTOR('',#15269,10.);
#4293=VECTOR('',#15272,10.);
#4294=VECTOR('',#15275,10.);
#4295=VECTOR('',#15276,10.);
#4296=VECTOR('',#15279,10.);
#4297=VECTOR('',#15280,10.);
#4298=VECTOR('',#15281,10.);
#4299=VECTOR('',#15282,10.);
#4300=VECTOR('',#15283,10.);
#4301=VECTOR('',#15284,10.);
#4302=VECTOR('',#15287,10.);
#4303=VECTOR('',#15290,10.);
#4304=VECTOR('',#15291,10.);
#4305=VECTOR('',#15294,10.);
#4306=VECTOR('',#15297,10.);
#4307=VECTOR('',#15300,10.);
#4308=VECTOR('',#15303,10.);
#4309=VECTOR('',#15306,10.);
#4310=VECTOR('',#15309,10.);
#4311=VECTOR('',#15310,10.);
#4312=VECTOR('',#15311,10.);
#4313=VECTOR('',#15314,10.);
#4314=VECTOR('',#15317,10.);
#4315=VECTOR('',#15320,10.);
#4316=VECTOR('',#15323,10.);
#4317=VECTOR('',#15326,10.);
#4318=VECTOR('',#15327,10.);
#4319=VECTOR('',#15328,10.);
#4320=VECTOR('',#15331,10.);
#4321=VECTOR('',#15334,10.);
#4322=VECTOR('',#15335,10.);
#4323=VECTOR('',#15338,10.);
#4324=VECTOR('',#15341,10.);
#4325=VECTOR('',#15344,10.);
#4326=VECTOR('',#15347,10.);
#4327=VECTOR('',#15350,10.);
#4328=VECTOR('',#15351,10.);
#4329=VECTOR('',#15354,10.);
#4330=VECTOR('',#15359,10.);
#4331=VECTOR('',#15362,10.);
#4332=VECTOR('',#15363,10.);
#4333=VECTOR('',#15366,10.);
#4334=VECTOR('',#15371,10.);
#4335=VECTOR('',#15374,10.);
#5584=VERTEX_POINT('',#18632);
#5585=VERTEX_POINT('',#18633);
#5586=VERTEX_POINT('',#18716);
#5587=VERTEX_POINT('',#18721);
#5588=VERTEX_POINT('',#18811);
#5589=VERTEX_POINT('',#18812);
#5590=VERTEX_POINT('',#18865);
#5591=VERTEX_POINT('',#18870);
#5592=VERTEX_POINT('',#18978);
#5593=VERTEX_POINT('',#18985);
#5594=VERTEX_POINT('',#18994);
#5595=VERTEX_POINT('',#18995);
#5596=VERTEX_POINT('',#18997);
#5597=VERTEX_POINT('',#18999);
#5598=VERTEX_POINT('',#19050);
#5599=VERTEX_POINT('',#19057);
#5600=VERTEX_POINT('',#19090);
#5601=VERTEX_POINT('',#19092);
#5602=VERTEX_POINT('',#19175);
#5603=VERTEX_POINT('',#19184);
#5604=VERTEX_POINT('',#19186);
#5605=VERTEX_POINT('',#19188);
#5606=VERTEX_POINT('',#19190);
#5607=VERTEX_POINT('',#19192);
#5608=VERTEX_POINT('',#19196);
#5609=VERTEX_POINT('',#19198);
#5610=VERTEX_POINT('',#19251);
#5611=VERTEX_POINT('',#19258);
#5612=VERTEX_POINT('',#19263);
#5613=VERTEX_POINT('',#19265);
#5614=VERTEX_POINT('',#19270);
#5615=VERTEX_POINT('',#19349);
#5616=VERTEX_POINT('',#19350);
#5617=VERTEX_POINT('',#19433);
#5618=VERTEX_POINT('',#19438);
#5619=VERTEX_POINT('',#19528);
#5620=VERTEX_POINT('',#19609);
#5621=VERTEX_POINT('',#19618);
#5622=VERTEX_POINT('',#19619);
#5623=VERTEX_POINT('',#19621);
#5624=VERTEX_POINT('',#19623);
#5625=VERTEX_POINT('',#19674);
#5626=VERTEX_POINT('',#19681);
#5627=VERTEX_POINT('',#19714);
#5628=VERTEX_POINT('',#19716);
#5629=VERTEX_POINT('',#19718);
#5630=VERTEX_POINT('',#19720);
#5631=VERTEX_POINT('',#19743);
#5632=VERTEX_POINT('',#19826);
#5633=VERTEX_POINT('',#19919);
#5634=VERTEX_POINT('',#19920);
#5635=VERTEX_POINT('',#19973);
#5636=VERTEX_POINT('',#19978);
#5637=VERTEX_POINT('',#20086);
#5638=VERTEX_POINT('',#20093);
#5639=VERTEX_POINT('',#20102);
#5640=VERTEX_POINT('',#20103);
#5641=VERTEX_POINT('',#20105);
#5642=VERTEX_POINT('',#20107);
#5643=VERTEX_POINT('',#20158);
#5644=VERTEX_POINT('',#20165);
#5645=VERTEX_POINT('',#20198);
#5646=VERTEX_POINT('',#20281);
#5647=VERTEX_POINT('',#20311);
#5648=VERTEX_POINT('',#20312);
#5649=VERTEX_POINT('',#20466);
#5650=VERTEX_POINT('',#20468);
#5651=VERTEX_POINT('',#20515);
#5652=VERTEX_POINT('',#20544);
#5653=VERTEX_POINT('',#20546);
#5654=VERTEX_POINT('',#20548);
#5655=VERTEX_POINT('',#20550);
#5656=VERTEX_POINT('',#20554);
#5657=VERTEX_POINT('',#20563);
#5658=VERTEX_POINT('',#20571);
#5659=VERTEX_POINT('',#20578);
#5660=VERTEX_POINT('',#20590);
#5661=VERTEX_POINT('',#20599);
#5662=VERTEX_POINT('',#20607);
#5663=VERTEX_POINT('',#20614);
#6831=EDGE_CURVE('',#5584,#5585,#88,.T.);
#6832=EDGE_CURVE('',#5586,#5585,#89,.T.);
#6833=EDGE_CURVE('',#5586,#5587,#90,.T.);
#6834=EDGE_CURVE('',#5587,#5584,#2977,.T.);
#6835=EDGE_CURVE('',#5588,#5589,#91,.T.);
#6836=EDGE_CURVE('',#5590,#5589,#92,.T.);
#6837=EDGE_CURVE('',#5590,#5591,#93,.T.);
#6838=EDGE_CURVE('',#5591,#5588,#2978,.T.);
#6839=EDGE_CURVE('',#5589,#5592,#94,.T.);
#6840=EDGE_CURVE('',#5592,#5593,#2979,.T.);
#6841=EDGE_CURVE('',#5593,#5590,#95,.T.);
#6842=EDGE_CURVE('',#5594,#5595,#2980,.T.);
#6843=EDGE_CURVE('',#5595,#5596,#807,.T.);
#6844=EDGE_CURVE('',#5596,#5597,#2981,.T.);
#6845=EDGE_CURVE('',#5597,#5594,#808,.T.);
#6846=EDGE_CURVE('',#5594,#5593,#96,.T.);
#6847=EDGE_CURVE('',#5592,#5595,#97,.T.);
#6848=EDGE_CURVE('',#5585,#5598,#98,.T.);
#6849=EDGE_CURVE('',#5598,#5599,#2982,.T.);
#6850=EDGE_CURVE('',#5599,#5586,#99,.T.);
#6851=EDGE_CURVE('',#5598,#5597,#100,.T.);
#6852=EDGE_CURVE('',#5596,#5599,#101,.T.);
#6853=EDGE_CURVE('',#5584,#5600,#2983,.T.);
#6854=EDGE_CURVE('',#5601,#5600,#102,.T.);
#6855=EDGE_CURVE('',#5602,#5601,#103,.T.);
#6856=EDGE_CURVE('',#5602,#5598,#2984,.T.);
#6857=EDGE_CURVE('',#5587,#5603,#2985,.T.);
#6858=EDGE_CURVE('',#5604,#5603,#2986,.T.);
#6859=EDGE_CURVE('',#5605,#5604,#2987,.T.);
#6860=EDGE_CURVE('',#5606,#5605,#2988,.T.);
#6861=EDGE_CURVE('',#5607,#5606,#2989,.T.);
#6862=EDGE_CURVE('',#5600,#5607,#2990,.T.);
#6863=EDGE_CURVE('',#5588,#5608,#2991,.T.);
#6864=EDGE_CURVE('',#5609,#5608,#104,.T.);
#6865=EDGE_CURVE('',#5610,#5609,#105,.T.);
#6866=EDGE_CURVE('',#5611,#5610,#106,.T.);
#6867=EDGE_CURVE('',#5612,#5611,#809,.T.);
#6868=EDGE_CURVE('',#5613,#5612,#107,.T.);
#6869=EDGE_CURVE('',#5614,#5613,#108,.T.);
#6870=EDGE_CURVE('',#5603,#5614,#109,.T.);
#6871=EDGE_CURVE('',#5615,#5616,#110,.T.);
#6872=EDGE_CURVE('',#5617,#5616,#111,.T.);
#6873=EDGE_CURVE('',#5617,#5618,#112,.T.);
#6874=EDGE_CURVE('',#5618,#5615,#2992,.T.);
#6875=EDGE_CURVE('',#5607,#5619,#113,.T.);
#6876=EDGE_CURVE('',#5601,#5619,#114,.T.);
#6877=EDGE_CURVE('',#5619,#5620,#115,.T.);
#6878=EDGE_CURVE('',#5620,#5602,#2993,.T.);
#6879=EDGE_CURVE('',#5621,#5622,#2994,.T.);
#6880=EDGE_CURVE('',#5622,#5623,#810,.T.);
#6881=EDGE_CURVE('',#5623,#5624,#2995,.T.);
#6882=EDGE_CURVE('',#5624,#5621,#811,.T.);
#6883=EDGE_CURVE('',#5621,#5602,#116,.T.);
#6884=EDGE_CURVE('',#5620,#5622,#117,.T.);
#6885=EDGE_CURVE('',#5616,#5625,#118,.T.);
#6886=EDGE_CURVE('',#5625,#5626,#2996,.T.);
#6887=EDGE_CURVE('',#5626,#5617,#119,.T.);
#6888=EDGE_CURVE('',#5625,#5624,#120,.T.);
#6889=EDGE_CURVE('',#5623,#5626,#121,.T.);
#6890=EDGE_CURVE('',#5627,#5625,#2997,.T.);
#6891=EDGE_CURVE('',#5628,#5627,#812,.T.);
#6892=EDGE_CURVE('',#5629,#5628,#2998,.T.);
#6893=EDGE_CURVE('',#5630,#5629,#813,.T.);
#6894=EDGE_CURVE('',#5593,#5630,#2999,.T.);
#6895=EDGE_CURVE('',#5605,#5631,#122,.T.);
#6896=EDGE_CURVE('',#5632,#5631,#123,.T.);
#6897=EDGE_CURVE('',#5632,#5606,#124,.T.);
#6898=EDGE_CURVE('',#5633,#5634,#125,.T.);
#6899=EDGE_CURVE('',#5635,#5634,#126,.T.);
#6900=EDGE_CURVE('',#5635,#5636,#127,.T.);
#6901=EDGE_CURVE('',#5636,#5633,#3000,.T.);
#6902=EDGE_CURVE('',#5634,#5637,#128,.T.);
#6903=EDGE_CURVE('',#5637,#5638,#3001,.T.);
#6904=EDGE_CURVE('',#5638,#5635,#129,.T.);
#6905=EDGE_CURVE('',#5639,#5640,#3002,.T.);
#6906=EDGE_CURVE('',#5640,#5641,#814,.T.);
#6907=EDGE_CURVE('',#5641,#5642,#3003,.T.);
#6908=EDGE_CURVE('',#5642,#5639,#815,.T.);
#6909=EDGE_CURVE('',#5641,#5638,#130,.T.);
#6910=EDGE_CURVE('',#5637,#5642,#131,.T.);
#6911=EDGE_CURVE('',#5631,#5643,#132,.T.);
#6912=EDGE_CURVE('',#5643,#5644,#3004,.T.);
#6913=EDGE_CURVE('',#5644,#5632,#133,.T.);
#6914=EDGE_CURVE('',#5643,#5640,#134,.T.);
#6915=EDGE_CURVE('',#5639,#5644,#135,.T.);
#6916=EDGE_CURVE('',#5645,#5604,#136,.T.);
#6917=EDGE_CURVE('',#5646,#5645,#137,.T.);
#6918=EDGE_CURVE('',#5646,#5643,#3005,.T.);
#6919=EDGE_CURVE('',#5618,#5633,#3006,.T.);
#6920=EDGE_CURVE('',#5647,#5648,#138,.T.);
#6921=EDGE_CURVE('',#5609,#5648,#139,.T.);
#6922=EDGE_CURVE('',#5608,#5647,#3007,.T.);
#6923=EDGE_CURVE('',#5645,#5614,#140,.T.);
#6924=EDGE_CURVE('',#5613,#5646,#3008,.T.);
#6925=EDGE_CURVE('',#5611,#5649,#3009,.T.);
#6926=EDGE_CURVE('',#5649,#5650,#816,.T.);
#6927=EDGE_CURVE('',#5650,#5612,#3010,.T.);
#6928=EDGE_CURVE('',#5650,#5646,#141,.T.);
#6929=EDGE_CURVE('',#5648,#5651,#142,.T.);
#6930=EDGE_CURVE('',#5651,#5610,#3011,.T.);
#6931=EDGE_CURVE('',#5651,#5649,#143,.T.);
#6932=EDGE_CURVE('',#5652,#5651,#3012,.T.);
#6933=EDGE_CURVE('',#5652,#5653,#817,.T.);
#6934=EDGE_CURVE('',#5654,#5653,#3013,.T.);
#6935=EDGE_CURVE('',#5654,#5655,#818,.T.);
#6936=EDGE_CURVE('',#5638,#5655,#3014,.T.);
#6937=EDGE_CURVE('',#5647,#5656,#3015,.T.);
#6938=EDGE_CURVE('',#5656,#5652,#144,.T.);
#6939=EDGE_CURVE('',#5657,#5656,#3016,.T.);
#6940=EDGE_CURVE('',#5630,#5657,#145,.T.);
#6941=EDGE_CURVE('',#5658,#5629,#146,.T.);
#6942=EDGE_CURVE('',#5658,#5659,#3017,.T.);
#6943=EDGE_CURVE('',#5653,#5659,#147,.T.);
#6944=EDGE_CURVE('',#5657,#5591,#3018,.T.);
#6945=EDGE_CURVE('',#5660,#5654,#148,.T.);
#6946=EDGE_CURVE('',#5659,#5660,#3019,.T.);
#6947=EDGE_CURVE('',#5661,#5660,#3020,.T.);
#6948=EDGE_CURVE('',#5628,#5661,#149,.T.);
#6949=EDGE_CURVE('',#5662,#5627,#150,.T.);
#6950=EDGE_CURVE('',#5662,#5663,#3021,.T.);
#6951=EDGE_CURVE('',#5655,#5663,#151,.T.);
#6952=EDGE_CURVE('',#5661,#5658,#3022,.T.);
#6953=EDGE_CURVE('',#5663,#5636,#3023,.T.);
#6954=EDGE_CURVE('',#5615,#5662,#3024,.T.);
#8909=ORIENTED_EDGE('',*,*,#6831,.T.);
#8910=ORIENTED_EDGE('',*,*,#6832,.F.);
#8911=ORIENTED_EDGE('',*,*,#6833,.T.);
#8912=ORIENTED_EDGE('',*,*,#6834,.T.);
#8913=ORIENTED_EDGE('',*,*,#6835,.T.);
#8914=ORIENTED_EDGE('',*,*,#6836,.F.);
#8915=ORIENTED_EDGE('',*,*,#6837,.T.);
#8916=ORIENTED_EDGE('',*,*,#6838,.T.);
#8917=ORIENTED_EDGE('',*,*,#6836,.T.);
#8918=ORIENTED_EDGE('',*,*,#6839,.T.);
#8919=ORIENTED_EDGE('',*,*,#6840,.T.);
#8920=ORIENTED_EDGE('',*,*,#6841,.T.);
#8921=ORIENTED_EDGE('',*,*,#6842,.T.);
#8922=ORIENTED_EDGE('',*,*,#6843,.T.);
#8923=ORIENTED_EDGE('',*,*,#6844,.T.);
#8924=ORIENTED_EDGE('',*,*,#6845,.T.);
#8925=ORIENTED_EDGE('',*,*,#6842,.F.);
#8926=ORIENTED_EDGE('',*,*,#6846,.T.);
#8927=ORIENTED_EDGE('',*,*,#6840,.F.);
#8928=ORIENTED_EDGE('',*,*,#6847,.T.);
#8929=ORIENTED_EDGE('',*,*,#6832,.T.);
#8930=ORIENTED_EDGE('',*,*,#6848,.T.);
#8931=ORIENTED_EDGE('',*,*,#6849,.T.);
#8932=ORIENTED_EDGE('',*,*,#6850,.T.);
#8933=ORIENTED_EDGE('',*,*,#6849,.F.);
#8934=ORIENTED_EDGE('',*,*,#6851,.T.);
#8935=ORIENTED_EDGE('',*,*,#6844,.F.);
#8936=ORIENTED_EDGE('',*,*,#6852,.T.);
#8937=ORIENTED_EDGE('',*,*,#6848,.F.);
#8938=ORIENTED_EDGE('',*,*,#6831,.F.);
#8939=ORIENTED_EDGE('',*,*,#6853,.T.);
#8940=ORIENTED_EDGE('',*,*,#6854,.F.);
#8941=ORIENTED_EDGE('',*,*,#6855,.F.);
#8942=ORIENTED_EDGE('',*,*,#6856,.T.);
#8943=ORIENTED_EDGE('',*,*,#6834,.F.);
#8944=ORIENTED_EDGE('',*,*,#6857,.T.);
#8945=ORIENTED_EDGE('',*,*,#6858,.F.);
#8946=ORIENTED_EDGE('',*,*,#6859,.F.);
#8947=ORIENTED_EDGE('',*,*,#6860,.F.);
#8948=ORIENTED_EDGE('',*,*,#6861,.F.);
#8949=ORIENTED_EDGE('',*,*,#6862,.F.);
#8950=ORIENTED_EDGE('',*,*,#6853,.F.);
#8951=ORIENTED_EDGE('',*,*,#6833,.F.);
#8952=ORIENTED_EDGE('',*,*,#6850,.F.);
#8953=ORIENTED_EDGE('',*,*,#6852,.F.);
#8954=ORIENTED_EDGE('',*,*,#6843,.F.);
#8955=ORIENTED_EDGE('',*,*,#6847,.F.);
#8956=ORIENTED_EDGE('',*,*,#6839,.F.);
#8957=ORIENTED_EDGE('',*,*,#6835,.F.);
#8958=ORIENTED_EDGE('',*,*,#6863,.T.);
#8959=ORIENTED_EDGE('',*,*,#6864,.F.);
#8960=ORIENTED_EDGE('',*,*,#6865,.F.);
#8961=ORIENTED_EDGE('',*,*,#6866,.F.);
#8962=ORIENTED_EDGE('',*,*,#6867,.F.);
#8963=ORIENTED_EDGE('',*,*,#6868,.F.);
#8964=ORIENTED_EDGE('',*,*,#6869,.F.);
#8965=ORIENTED_EDGE('',*,*,#6870,.F.);
#8966=ORIENTED_EDGE('',*,*,#6857,.F.);
#8967=ORIENTED_EDGE('',*,*,#6871,.T.);
#8968=ORIENTED_EDGE('',*,*,#6872,.F.);
#8969=ORIENTED_EDGE('',*,*,#6873,.T.);
#8970=ORIENTED_EDGE('',*,*,#6874,.T.);
#8971=ORIENTED_EDGE('',*,*,#6875,.T.);
#8972=ORIENTED_EDGE('',*,*,#6876,.F.);
#8973=ORIENTED_EDGE('',*,*,#6854,.T.);
#8974=ORIENTED_EDGE('',*,*,#6862,.T.);
#8975=ORIENTED_EDGE('',*,*,#6876,.T.);
#8976=ORIENTED_EDGE('',*,*,#6877,.T.);
#8977=ORIENTED_EDGE('',*,*,#6878,.T.);
#8978=ORIENTED_EDGE('',*,*,#6855,.T.);
#8979=ORIENTED_EDGE('',*,*,#6879,.T.);
#8980=ORIENTED_EDGE('',*,*,#6880,.T.);
#8981=ORIENTED_EDGE('',*,*,#6881,.T.);
#8982=ORIENTED_EDGE('',*,*,#6882,.T.);
#8983=ORIENTED_EDGE('',*,*,#6879,.F.);
#8984=ORIENTED_EDGE('',*,*,#6883,.T.);
#8985=ORIENTED_EDGE('',*,*,#6878,.F.);
#8986=ORIENTED_EDGE('',*,*,#6884,.T.);
#8987=ORIENTED_EDGE('',*,*,#6872,.T.);
#8988=ORIENTED_EDGE('',*,*,#6885,.T.);
#8989=ORIENTED_EDGE('',*,*,#6886,.T.);
#8990=ORIENTED_EDGE('',*,*,#6887,.T.);
#8991=ORIENTED_EDGE('',*,*,#6886,.F.);
#8992=ORIENTED_EDGE('',*,*,#6888,.T.);
#8993=ORIENTED_EDGE('',*,*,#6881,.F.);
#8994=ORIENTED_EDGE('',*,*,#6889,.T.);
#8995=ORIENTED_EDGE('',*,*,#6851,.F.);
#8996=ORIENTED_EDGE('',*,*,#6856,.F.);
#8997=ORIENTED_EDGE('',*,*,#6883,.F.);
#8998=ORIENTED_EDGE('',*,*,#6882,.F.);
#8999=ORIENTED_EDGE('',*,*,#6888,.F.);
#9000=ORIENTED_EDGE('',*,*,#6890,.F.);
#9001=ORIENTED_EDGE('',*,*,#6891,.F.);
#9002=ORIENTED_EDGE('',*,*,#6892,.F.);
#9003=ORIENTED_EDGE('',*,*,#6893,.F.);
#9004=ORIENTED_EDGE('',*,*,#6894,.F.);
#9005=ORIENTED_EDGE('',*,*,#6846,.F.);
#9006=ORIENTED_EDGE('',*,*,#6845,.F.);
#9007=ORIENTED_EDGE('',*,*,#6895,.T.);
#9008=ORIENTED_EDGE('',*,*,#6896,.F.);
#9009=ORIENTED_EDGE('',*,*,#6897,.T.);
#9010=ORIENTED_EDGE('',*,*,#6860,.T.);
#9011=ORIENTED_EDGE('',*,*,#6898,.T.);
#9012=ORIENTED_EDGE('',*,*,#6899,.F.);
#9013=ORIENTED_EDGE('',*,*,#6900,.T.);
#9014=ORIENTED_EDGE('',*,*,#6901,.T.);
#9015=ORIENTED_EDGE('',*,*,#6899,.T.);
#9016=ORIENTED_EDGE('',*,*,#6902,.T.);
#9017=ORIENTED_EDGE('',*,*,#6903,.T.);
#9018=ORIENTED_EDGE('',*,*,#6904,.T.);
#9019=ORIENTED_EDGE('',*,*,#6905,.T.);
#9020=ORIENTED_EDGE('',*,*,#6906,.T.);
#9021=ORIENTED_EDGE('',*,*,#6907,.T.);
#9022=ORIENTED_EDGE('',*,*,#6908,.T.);
#9023=ORIENTED_EDGE('',*,*,#6907,.F.);
#9024=ORIENTED_EDGE('',*,*,#6909,.T.);
#9025=ORIENTED_EDGE('',*,*,#6903,.F.);
#9026=ORIENTED_EDGE('',*,*,#6910,.T.);
#9027=ORIENTED_EDGE('',*,*,#6896,.T.);
#9028=ORIENTED_EDGE('',*,*,#6911,.T.);
#9029=ORIENTED_EDGE('',*,*,#6912,.T.);
#9030=ORIENTED_EDGE('',*,*,#6913,.T.);
#9031=ORIENTED_EDGE('',*,*,#6912,.F.);
#9032=ORIENTED_EDGE('',*,*,#6914,.T.);
#9033=ORIENTED_EDGE('',*,*,#6905,.F.);
#9034=ORIENTED_EDGE('',*,*,#6915,.T.);
#9035=ORIENTED_EDGE('',*,*,#6911,.F.);
#9036=ORIENTED_EDGE('',*,*,#6895,.F.);
#9037=ORIENTED_EDGE('',*,*,#6859,.T.);
#9038=ORIENTED_EDGE('',*,*,#6916,.F.);
#9039=ORIENTED_EDGE('',*,*,#6917,.F.);
#9040=ORIENTED_EDGE('',*,*,#6918,.T.);
#9041=ORIENTED_EDGE('',*,*,#6875,.F.);
#9042=ORIENTED_EDGE('',*,*,#6861,.T.);
#9043=ORIENTED_EDGE('',*,*,#6897,.F.);
#9044=ORIENTED_EDGE('',*,*,#6913,.F.);
#9045=ORIENTED_EDGE('',*,*,#6915,.F.);
#9046=ORIENTED_EDGE('',*,*,#6908,.F.);
#9047=ORIENTED_EDGE('',*,*,#6910,.F.);
#9048=ORIENTED_EDGE('',*,*,#6902,.F.);
#9049=ORIENTED_EDGE('',*,*,#6898,.F.);
#9050=ORIENTED_EDGE('',*,*,#6919,.F.);
#9051=ORIENTED_EDGE('',*,*,#6873,.F.);
#9052=ORIENTED_EDGE('',*,*,#6887,.F.);
#9053=ORIENTED_EDGE('',*,*,#6889,.F.);
#9054=ORIENTED_EDGE('',*,*,#6880,.F.);
#9055=ORIENTED_EDGE('',*,*,#6884,.F.);
#9056=ORIENTED_EDGE('',*,*,#6877,.F.);
#9057=ORIENTED_EDGE('',*,*,#6920,.T.);
#9058=ORIENTED_EDGE('',*,*,#6921,.F.);
#9059=ORIENTED_EDGE('',*,*,#6864,.T.);
#9060=ORIENTED_EDGE('',*,*,#6922,.T.);
#9061=ORIENTED_EDGE('',*,*,#6870,.T.);
#9062=ORIENTED_EDGE('',*,*,#6923,.F.);
#9063=ORIENTED_EDGE('',*,*,#6916,.T.);
#9064=ORIENTED_EDGE('',*,*,#6858,.T.);
#9065=ORIENTED_EDGE('',*,*,#6923,.T.);
#9066=ORIENTED_EDGE('',*,*,#6869,.T.);
#9067=ORIENTED_EDGE('',*,*,#6924,.T.);
#9068=ORIENTED_EDGE('',*,*,#6917,.T.);
#9069=ORIENTED_EDGE('',*,*,#6925,.T.);
#9070=ORIENTED_EDGE('',*,*,#6926,.T.);
#9071=ORIENTED_EDGE('',*,*,#6927,.T.);
#9072=ORIENTED_EDGE('',*,*,#6867,.T.);
#9073=ORIENTED_EDGE('',*,*,#6927,.F.);
#9074=ORIENTED_EDGE('',*,*,#6928,.T.);
#9075=ORIENTED_EDGE('',*,*,#6924,.F.);
#9076=ORIENTED_EDGE('',*,*,#6868,.T.);
#9077=ORIENTED_EDGE('',*,*,#6921,.T.);
#9078=ORIENTED_EDGE('',*,*,#6929,.T.);
#9079=ORIENTED_EDGE('',*,*,#6930,.T.);
#9080=ORIENTED_EDGE('',*,*,#6865,.T.);
#9081=ORIENTED_EDGE('',*,*,#6930,.F.);
#9082=ORIENTED_EDGE('',*,*,#6931,.T.);
#9083=ORIENTED_EDGE('',*,*,#6925,.F.);
#9084=ORIENTED_EDGE('',*,*,#6866,.T.);
#9085=ORIENTED_EDGE('',*,*,#6914,.F.);
#9086=ORIENTED_EDGE('',*,*,#6918,.F.);
#9087=ORIENTED_EDGE('',*,*,#6928,.F.);
#9088=ORIENTED_EDGE('',*,*,#6926,.F.);
#9089=ORIENTED_EDGE('',*,*,#6931,.F.);
#9090=ORIENTED_EDGE('',*,*,#6932,.F.);
#9091=ORIENTED_EDGE('',*,*,#6933,.T.);
#9092=ORIENTED_EDGE('',*,*,#6934,.F.);
#9093=ORIENTED_EDGE('',*,*,#6935,.T.);
#9094=ORIENTED_EDGE('',*,*,#6936,.F.);
#9095=ORIENTED_EDGE('',*,*,#6909,.F.);
#9096=ORIENTED_EDGE('',*,*,#6906,.F.);
#9097=ORIENTED_EDGE('',*,*,#6920,.F.);
#9098=ORIENTED_EDGE('',*,*,#6937,.T.);
#9099=ORIENTED_EDGE('',*,*,#6938,.T.);
#9100=ORIENTED_EDGE('',*,*,#6932,.T.);
#9101=ORIENTED_EDGE('',*,*,#6929,.F.);
#9102=ORIENTED_EDGE('',*,*,#6938,.F.);
#9103=ORIENTED_EDGE('',*,*,#6939,.F.);
#9104=ORIENTED_EDGE('',*,*,#6940,.F.);
#9105=ORIENTED_EDGE('',*,*,#6893,.T.);
#9106=ORIENTED_EDGE('',*,*,#6941,.F.);
#9107=ORIENTED_EDGE('',*,*,#6942,.T.);
#9108=ORIENTED_EDGE('',*,*,#6943,.F.);
#9109=ORIENTED_EDGE('',*,*,#6933,.F.);
#9110=ORIENTED_EDGE('',*,*,#6838,.F.);
#9111=ORIENTED_EDGE('',*,*,#6944,.F.);
#9112=ORIENTED_EDGE('',*,*,#6939,.T.);
#9113=ORIENTED_EDGE('',*,*,#6937,.F.);
#9114=ORIENTED_EDGE('',*,*,#6922,.F.);
#9115=ORIENTED_EDGE('',*,*,#6863,.F.);
#9116=ORIENTED_EDGE('',*,*,#6841,.F.);
#9117=ORIENTED_EDGE('',*,*,#6894,.T.);
#9118=ORIENTED_EDGE('',*,*,#6940,.T.);
#9119=ORIENTED_EDGE('',*,*,#6944,.T.);
#9120=ORIENTED_EDGE('',*,*,#6837,.F.);
#9121=ORIENTED_EDGE('',*,*,#6945,.T.);
#9122=ORIENTED_EDGE('',*,*,#6934,.T.);
#9123=ORIENTED_EDGE('',*,*,#6943,.T.);
#9124=ORIENTED_EDGE('',*,*,#6946,.T.);
#9125=ORIENTED_EDGE('',*,*,#6945,.F.);
#9126=ORIENTED_EDGE('',*,*,#6947,.F.);
#9127=ORIENTED_EDGE('',*,*,#6948,.F.);
#9128=ORIENTED_EDGE('',*,*,#6891,.T.);
#9129=ORIENTED_EDGE('',*,*,#6949,.F.);
#9130=ORIENTED_EDGE('',*,*,#6950,.T.);
#9131=ORIENTED_EDGE('',*,*,#6951,.F.);
#9132=ORIENTED_EDGE('',*,*,#6935,.F.);
#9133=ORIENTED_EDGE('',*,*,#6946,.F.);
#9134=ORIENTED_EDGE('',*,*,#6942,.F.);
#9135=ORIENTED_EDGE('',*,*,#6952,.F.);
#9136=ORIENTED_EDGE('',*,*,#6947,.T.);
#9137=ORIENTED_EDGE('',*,*,#6948,.T.);
#9138=ORIENTED_EDGE('',*,*,#6952,.T.);
#9139=ORIENTED_EDGE('',*,*,#6941,.T.);
#9140=ORIENTED_EDGE('',*,*,#6892,.T.);
#9141=ORIENTED_EDGE('',*,*,#6904,.F.);
#9142=ORIENTED_EDGE('',*,*,#6936,.T.);
#9143=ORIENTED_EDGE('',*,*,#6951,.T.);
#9144=ORIENTED_EDGE('',*,*,#6953,.T.);
#9145=ORIENTED_EDGE('',*,*,#6900,.F.);
#9146=ORIENTED_EDGE('',*,*,#6874,.F.);
#9147=ORIENTED_EDGE('',*,*,#6919,.T.);
#9148=ORIENTED_EDGE('',*,*,#6901,.F.);
#9149=ORIENTED_EDGE('',*,*,#6953,.F.);
#9150=ORIENTED_EDGE('',*,*,#6950,.F.);
#9151=ORIENTED_EDGE('',*,*,#6954,.F.);
#9152=ORIENTED_EDGE('',*,*,#6871,.F.);
#9153=ORIENTED_EDGE('',*,*,#6954,.T.);
#9154=ORIENTED_EDGE('',*,*,#6949,.T.);
#9155=ORIENTED_EDGE('',*,*,#6890,.T.);
#9156=ORIENTED_EDGE('',*,*,#6885,.F.);
#12631=PLANE('',#14065);
#12632=PLANE('',#14071);
#12633=PLANE('',#14081);
#12634=PLANE('',#14086);
#12635=PLANE('',#14090);
#12636=PLANE('',#14093);
#13056=ADVANCED_FACE('',(#1293),#407,.T.);
#13057=ADVANCED_FACE('',(#1294),#408,.T.);
#13058=ADVANCED_FACE('',(#1295),#409,.T.);
#13059=ADVANCED_FACE('',(#1296),#1113,.T.);
#13060=ADVANCED_FACE('',(#1297),#410,.T.);
#13061=ADVANCED_FACE('',(#1298),#411,.T.);
#13062=ADVANCED_FACE('',(#1299),#412,.T.);
#13063=ADVANCED_FACE('',(#1300),#656,.T.);
#13064=ADVANCED_FACE('',(#1301),#12631,.T.);
#13065=ADVANCED_FACE('',(#1302),#657,.T.);
#13066=ADVANCED_FACE('',(#1303),#413,.T.);
#13067=ADVANCED_FACE('',(#1304),#414,.T.);
#13068=ADVANCED_FACE('',(#1305),#415,.T.);
#13069=ADVANCED_FACE('',(#1306),#1114,.T.);
#13070=ADVANCED_FACE('',(#1307),#416,.T.);
#13071=ADVANCED_FACE('',(#1308),#417,.T.);
#13072=ADVANCED_FACE('',(#1309),#418,.T.);
#13073=ADVANCED_FACE('',(#1310),#12632,.F.);
#13074=ADVANCED_FACE('',(#1311),#419,.T.);
#13075=ADVANCED_FACE('',(#1312),#420,.T.);
#13076=ADVANCED_FACE('',(#1313),#421,.T.);
#13077=ADVANCED_FACE('',(#1314),#1115,.T.);
#13078=ADVANCED_FACE('',(#1315),#422,.T.);
#13079=ADVANCED_FACE('',(#1316),#423,.T.);
#13080=ADVANCED_FACE('',(#1317),#424,.T.);
#13081=ADVANCED_FACE('',(#1318),#658,.T.);
#13082=ADVANCED_FACE('',(#1319),#659,.T.);
#13083=ADVANCED_FACE('',(#1320),#425,.T.);
#13084=ADVANCED_FACE('',(#1321),#426,.T.);
#13085=ADVANCED_FACE('',(#1322),#427,.T.);
#13086=ADVANCED_FACE('',(#1323),#1116,.T.);
#13087=ADVANCED_FACE('',(#1324),#428,.T.);
#13088=ADVANCED_FACE('',(#1325),#429,.T.);
#13089=ADVANCED_FACE('',(#1326),#430,.T.);
#13090=ADVANCED_FACE('',(#1327),#12633,.T.);
#13091=ADVANCED_FACE('',(#1328),#660,.T.);
#13092=ADVANCED_FACE('',(#1329),#661,.T.);
#13093=ADVANCED_FACE('',(#1330),#12634,.T.);
#13094=ADVANCED_FACE('',(#1331),#662,.T.);
#13095=ADVANCED_FACE('',(#1332),#663,.T.);
#13096=ADVANCED_FACE('',(#1333),#664,.T.);
#13097=ADVANCED_FACE('',(#1334),#12635,.T.);
#13098=ADVANCED_FACE('',(#1335),#665,.T.);
#13099=ADVANCED_FACE('',(#1336),#666,.T.);
#13100=ADVANCED_FACE('',(#1337),#12636,.T.);
#13101=ADVANCED_FACE('',(#1338),#667,.T.);
#13805=CLOSED_SHELL('',(#13056,#13057,#13058,#13059,#13060,#13061,#13062,
#13063,#13064,#13065,#13066,#13067,#13068,#13069,#13070,#13071,#13072,#13073,
#13074,#13075,#13076,#13077,#13078,#13079,#13080,#13081,#13082,#13083,#13084,
#13085,#13086,#13087,#13088,#13089,#13090,#13091,#13092,#13093,#13094,#13095,
#13096,#13097,#13098,#13099,#13100,#13101));
#14060=AXIS2_PLACEMENT_3D('',#18611,#15259,#15260);
#14061=AXIS2_PLACEMENT_3D('',#18993,#15264,#15265);
#14062=AXIS2_PLACEMENT_3D('',#18998,#15267,#15268);
#14063=AXIS2_PLACEMENT_3D('',#19001,#15270,#15271);
#14064=AXIS2_PLACEMENT_3D('',#19089,#15273,#15274);
#14065=AXIS2_PLACEMENT_3D('',#19183,#15277,#15278);
#14066=AXIS2_PLACEMENT_3D('',#19195,#15285,#15286);
#14067=AXIS2_PLACEMENT_3D('',#19264,#15288,#15289);
#14068=AXIS2_PLACEMENT_3D('',#19617,#15292,#15293);
#14069=AXIS2_PLACEMENT_3D('',#19622,#15295,#15296);
#14070=AXIS2_PLACEMENT_3D('',#19625,#15298,#15299);
#14071=AXIS2_PLACEMENT_3D('',#19713,#15301,#15302);
#14072=AXIS2_PLACEMENT_3D('',#19717,#15304,#15305);
#14073=AXIS2_PLACEMENT_3D('',#19721,#15307,#15308);
#14074=AXIS2_PLACEMENT_3D('',#20101,#15312,#15313);
#14075=AXIS2_PLACEMENT_3D('',#20106,#15315,#15316);
#14076=AXIS2_PLACEMENT_3D('',#20109,#15318,#15319);
#14077=AXIS2_PLACEMENT_3D('',#20197,#15321,#15322);
#14078=AXIS2_PLACEMENT_3D('',#20289,#15324,#15325);
#14079=AXIS2_PLACEMENT_3D('',#20465,#15329,#15330);
#14080=AXIS2_PLACEMENT_3D('',#20469,#15332,#15333);
#14081=AXIS2_PLACEMENT_3D('',#20543,#15336,#15337);
#14082=AXIS2_PLACEMENT_3D('',#20547,#15339,#15340);
#14083=AXIS2_PLACEMENT_3D('',#20551,#15342,#15343);
#14084=AXIS2_PLACEMENT_3D('',#20553,#15345,#15346);
#14085=AXIS2_PLACEMENT_3D('',#20562,#15348,#15349);
#14086=AXIS2_PLACEMENT_3D('',#20586,#15352,#15353);
#14087=AXIS2_PLACEMENT_3D('',#20588,#15355,#15356);
#14088=AXIS2_PLACEMENT_3D('',#20589,#15357,#15358);
#14089=AXIS2_PLACEMENT_3D('',#20598,#15360,#15361);
#14090=AXIS2_PLACEMENT_3D('',#20622,#15364,#15365);
#14091=AXIS2_PLACEMENT_3D('',#20624,#15367,#15368);
#14092=AXIS2_PLACEMENT_3D('',#20625,#15369,#15370);
#14093=AXIS2_PLACEMENT_3D('',#20627,#15372,#15373);
#14094=AXIS2_PLACEMENT_3D('',#20629,#15375,#15376);
#15259=DIRECTION('axis',(0.,0.,1.));
#15260=DIRECTION('refdir',(1.,0.,0.));
#15261=DIRECTION('',(-0.342997170284919,8.94256168307049E-16,0.93933643662776));
#15262=DIRECTION('',(0.342997170285,-0.939336436627731,0.));
#15263=DIRECTION('',(-0.737980838656753,0.364238207643154,0.568079932640097));
#15264=DIRECTION('center_axis',(1.,0.,0.));
#15265=DIRECTION('ref_axis',(0.,-1.,0.));
#15266=DIRECTION('',(0.707106781186544,-0.352766841475276,-0.612825877028347));
#15267=DIRECTION('center_axis',(-1.,0.,0.));
#15268=DIRECTION('ref_axis',(0.,-1.,0.));
#15269=DIRECTION('',(-0.707106781186552,0.612825877028345,0.352766841475263));
#15270=DIRECTION('center_axis',(1.,0.,0.));
#15271=DIRECTION('ref_axis',(0.,-1.,0.));
#15272=DIRECTION('',(0.737980838656762,-0.568079932640111,-0.364238207643115));
#15273=DIRECTION('center_axis',(0.,0.,-1.));
#15274=DIRECTION('ref_axis',(-0.70710678118654,-0.707106781186555,0.));
#15275=DIRECTION('',(0.,0.,1.));
#15276=DIRECTION('',(0.,0.,-1.));
#15277=DIRECTION('center_axis',(0.,-1.,0.));
#15278=DIRECTION('ref_axis',(0.,0.,-1.));
#15279=DIRECTION('',(1.,0.,0.));
#15280=DIRECTION('',(-0.342997170285006,-8.94256168307127E-16,-0.939336436627728));
#15281=DIRECTION('',(0.,0.,-1.));
#15282=DIRECTION('',(0.34299717028493,-2.68276850492124E-15,-0.939336436627756));
#15283=DIRECTION('',(1.,0.,0.));
#15284=DIRECTION('',(0.342997170285008,2.6827685049214E-15,0.939336436627727));
#15285=DIRECTION('center_axis',(1.,0.,0.));
#15286=DIRECTION('ref_axis',(0.,-1.,0.));
#15287=DIRECTION('',(1.,0.,0.));
#15288=DIRECTION('center_axis',(1.,0.,0.));
#15289=DIRECTION('ref_axis',(0.,-1.,0.));
#15290=DIRECTION('',(-0.342997170284998,0.939336436627731,0.));
#15291=DIRECTION('',(-0.737980838656755,0.568079932640103,-0.364238207643142));
#15292=DIRECTION('center_axis',(1.,0.,0.));
#15293=DIRECTION('ref_axis',(0.,-1.29526019539602E-15,1.));
#15294=DIRECTION('',(0.707106781186544,-0.612825877028338,0.352766841475291));
#15295=DIRECTION('center_axis',(-1.,0.,0.));
#15296=DIRECTION('ref_axis',(0.,-1.29526019539602E-15,1.));
#15297=DIRECTION('',(-0.707106781186543,0.352766841475279,-0.612825877028346));
#15298=DIRECTION('center_axis',(1.,0.,0.));
#15299=DIRECTION('ref_axis',(0.,-1.29526019539601E-15,1.));
#15300=DIRECTION('',(0.73798083899629,-0.364238207417434,0.568079932343738));
#15301=DIRECTION('center_axis',(1.,0.,0.));
#15302=DIRECTION('ref_axis',(0.,0.,-1.));
#15303=DIRECTION('',(0.,-1.,0.));
#15304=DIRECTION('center_axis',(1.,0.,0.));
#15305=DIRECTION('ref_axis',(0.,1.,-3.7007434154172E-15));
#15306=DIRECTION('',(0.,0.,1.));
#15307=DIRECTION('center_axis',(1.,0.,0.));
#15308=DIRECTION('ref_axis',(0.,-2.96059473233375E-15,-1.));
#15309=DIRECTION('',(0.,1.,0.));
#15310=DIRECTION('',(-0.342997170285007,-0.939336436627728,0.));
#15311=DIRECTION('',(0.737980838656857,0.364238207643107,-0.568079932639993));
#15312=DIRECTION('center_axis',(-1.,0.,0.));
#15313=DIRECTION('ref_axis',(0.,-1.29526019539602E-15,1.));
#15314=DIRECTION('',(0.707106781186544,0.612825877028338,-0.352766841475291));
#15315=DIRECTION('center_axis',(-1.,0.,0.));
#15316=DIRECTION('ref_axis',(0.,-1.29526019539601E-15,1.));
#15317=DIRECTION('',(-0.707106781186543,-0.352766841475279,0.612825877028346));
#15318=DIRECTION('center_axis',(1.,0.,0.));
#15319=DIRECTION('ref_axis',(0.,-1.29526019539602E-15,1.));
#15320=DIRECTION('',(-0.737980838996349,-0.568079932343716,0.364238207417348));
#15321=DIRECTION('center_axis',(0.,0.,-1.));
#15322=DIRECTION('ref_axis',(0.70710678118654,-0.707106781186555,0.));
#15323=DIRECTION('',(0.,0.,1.));
#15324=DIRECTION('center_axis',(1.,0.,0.));
#15325=DIRECTION('ref_axis',(0.,-1.29526019539602E-15,1.));
#15326=DIRECTION('',(1.,0.,0.));
#15327=DIRECTION('',(0.342997170285021,0.939336436627723,0.));
#15328=DIRECTION('',(0.737980838996329,0.568079932343672,0.364238207417458));
#15329=DIRECTION('center_axis',(-1.,0.,0.));
#15330=DIRECTION('ref_axis',(0.,-1.,0.));
#15331=DIRECTION('',(0.707106781186544,0.352766841475276,0.612825877028347));
#15332=DIRECTION('center_axis',(-1.,0.,0.));
#15333=DIRECTION('ref_axis',(0.,-1.,0.));
#15334=DIRECTION('',(-0.707106781186552,-0.612825877028345,-0.352766841475263));
#15335=DIRECTION('',(-0.737980838656747,-0.364238207643175,-0.568079932640092));
#15336=DIRECTION('center_axis',(1.,0.,0.));
#15337=DIRECTION('ref_axis',(0.,0.,-1.));
#15338=DIRECTION('',(0.,-1.,0.));
#15339=DIRECTION('center_axis',(1.,0.,0.));
#15340=DIRECTION('ref_axis',(0.,-2.96059473233375E-15,-1.));
#15341=DIRECTION('',(0.,0.,-1.));
#15342=DIRECTION('center_axis',(1.,0.,0.));
#15343=DIRECTION('ref_axis',(0.,1.,-3.7007434154172E-15));
#15344=DIRECTION('',(0.,1.,0.));
#15345=DIRECTION('center_axis',(0.,1.,0.));
#15346=DIRECTION('ref_axis',(0.707106781186532,0.,-0.707106781186563));
#15347=DIRECTION('',(0.,1.,0.));
#15348=DIRECTION('center_axis',(1.,0.,0.));
#15349=DIRECTION('ref_axis',(0.,-2.96059473233375E-15,-1.));
#15350=DIRECTION('',(1.,0.,0.));
#15351=DIRECTION('',(1.,0.,0.));
#15352=DIRECTION('center_axis',(0.,0.,-1.));
#15353=DIRECTION('ref_axis',(0.,1.,0.));
#15354=DIRECTION('',(0.,-1.,0.));
#15355=DIRECTION('center_axis',(0.,1.,0.));
#15356=DIRECTION('ref_axis',(-0.707106781186532,0.,-0.707106781186563));
#15357=DIRECTION('center_axis',(0.,0.,1.));
#15358=DIRECTION('ref_axis',(0.707106781186532,0.707106781186563,0.));
#15359=DIRECTION('',(0.,0.,1.));
#15360=DIRECTION('center_axis',(1.,0.,0.));
#15361=DIRECTION('ref_axis',(0.,1.,-3.7007434154172E-15));
#15362=DIRECTION('',(1.,0.,0.));
#15363=DIRECTION('',(1.,0.,0.));
#15364=DIRECTION('center_axis',(0.,1.,0.));
#15365=DIRECTION('ref_axis',(0.,0.,1.));
#15366=DIRECTION('',(0.,0.,-1.));
#15367=DIRECTION('center_axis',(0.,0.,1.));
#15368=DIRECTION('ref_axis',(-0.707106781186532,0.707106781186563,0.));
#15369=DIRECTION('center_axis',(0.,-1.,0.));
#15370=DIRECTION('ref_axis',(0.70710678118654,0.,0.707106781186555));
#15371=DIRECTION('',(0.,-1.,0.));
#15372=DIRECTION('center_axis',(0.,0.,1.));
#15373=DIRECTION('ref_axis',(0.,-1.,0.));
#15374=DIRECTION('',(0.,1.,0.));
#15375=DIRECTION('center_axis',(0.,-1.,0.));
#15376=DIRECTION('ref_axis',(-0.70710678118654,0.,0.707106781186555));
#18611=CARTESIAN_POINT('',(0.,0.,0.));
#18612=CARTESIAN_POINT('Ctrl Pts',(178.412949735578,0.0221746991903159,
-101.882758090243));
#18613=CARTESIAN_POINT('Ctrl Pts',(178.423188588538,0.0197124751515442,
-101.853918449636));
#18614=CARTESIAN_POINT('Ctrl Pts',(178.514954119049,-0.000380689216689832,
-101.59747251699));
#18615=CARTESIAN_POINT('Ctrl Pts',(178.592152319935,2.07285186112207E-16,
-101.38857532093));
#18616=CARTESIAN_POINT('Ctrl Pts',(178.6,5.55111512312591E-16,-101.366904810515));
#18617=CARTESIAN_POINT('Ctrl Pts',(178.537808007848,0.014917453309238,-101.928351016583));
#18618=CARTESIAN_POINT('Ctrl Pts',(178.545154918172,0.0138762567563856,
-101.907795776369));
#18619=CARTESIAN_POINT('Ctrl Pts',(178.609866781544,-0.0024252187702473,
-101.725953735215));
#18620=CARTESIAN_POINT('Ctrl Pts',(178.665385999329,1.38099875338694E-16,
-101.576687138619));
#18621=CARTESIAN_POINT('Ctrl Pts',(178.670972086323,3.70074341541732E-16,
-101.561269873677));
#18622=CARTESIAN_POINT('Ctrl Pts',(178.662666280119,0.00766020742816023,
-101.973943942923));
#18623=CARTESIAN_POINT('Ctrl Pts',(178.667057936009,0.00742672667316728,
-101.961748861519));
#18624=CARTESIAN_POINT('Ctrl Pts',(178.706720397631,0.00233113595076795,
-101.85253791136));
#18625=CARTESIAN_POINT('Ctrl Pts',(178.738619678723,6.91866932068973E-17,
-101.764798956307));
#18626=CARTESIAN_POINT('Ctrl Pts',(178.741944172646,1.85037170770872E-16,
-101.755634936838));
#18627=CARTESIAN_POINT('Ctrl Pts',(178.787524552389,0.000402961547082414,
-102.019536869264));
#18628=CARTESIAN_POINT('Ctrl Pts',(178.788941666476,0.000357983627884323,
-102.015656202882));
#18629=CARTESIAN_POINT('Ctrl Pts',(178.801571117716,-7.9890588520116E-6,
-101.981070701652));
#18630=CARTESIAN_POINT('Ctrl Pts',(178.811853358117,1.27573599516211E-29,
-101.952910773995));
#18631=CARTESIAN_POINT('Ctrl Pts',(178.812916258969,1.27573599516211E-29,
-101.95));
#18632=CARTESIAN_POINT('',(178.6,5.55111512312578E-16,-101.366904810515));
#18633=CARTESIAN_POINT('',(178.412949735578,0.0221746991903159,-101.882758090243));
#18634=CARTESIAN_POINT('Ctrl Pts',(178.6,4.44089209850063E-16,-101.366904810515));
#18635=CARTESIAN_POINT('Ctrl Pts',(178.59945852697,4.20005404597354E-16,
-101.368400029082));
#18636=CARTESIAN_POINT('Ctrl Pts',(178.598915538305,5.09286916248376E-7,
-101.369899384534));
#18637=CARTESIAN_POINT('Ctrl Pts',(178.598314541834,1.77548273883055E-6,
-101.37155677101));
#18638=CARTESIAN_POINT('Ctrl Pts',(178.597685600891,3.1005527405874E-6,
-101.373291220818));
#18639=CARTESIAN_POINT('Ctrl Pts',(178.596993140289,5.24993586700169E-6,
-101.375198716009));
#18640=CARTESIAN_POINT('Ctrl Pts',(178.596192315107,9.06159147229246E-6,
-101.377401328991));
#18641=CARTESIAN_POINT('Ctrl Pts',(178.595361925554,1.30139634384334E-5,
-101.379685256686));
#18642=CARTESIAN_POINT('Ctrl Pts',(178.594415090726,1.8748033103421E-5,
-101.382286305868));
#18643=CARTESIAN_POINT('Ctrl Pts',(178.593322100849,2.78719461983545E-5,
-101.385285246245));
#18644=CARTESIAN_POINT('Ctrl Pts',(178.592179791908,3.7407558304085E-5,
-101.388419508032));
#18645=CARTESIAN_POINT('Ctrl Pts',(178.590877924042,5.06497810078656E-5,
-101.391988146604));
#18646=CARTESIAN_POINT('Ctrl Pts',(178.589403202399,7.01856533839029E-5,
-101.396027187129));
#18647=CARTESIAN_POINT('Ctrl Pts',(178.587842980484,9.0854161485207E-5,
-101.400300400026));
#18648=CARTESIAN_POINT('Ctrl Pts',(178.586089389774,0.000118592479514606,
-101.405099836938));
#18649=CARTESIAN_POINT('Ctrl Pts',(178.584147820027,0.000157072676082226,
-101.410410677723));
#18650=CARTESIAN_POINT('Ctrl Pts',(178.5820491216,0.000198667024222329,
-101.41615131785));
#18651=CARTESIAN_POINT('Ctrl Pts',(178.579730945858,0.000252874493260704,
-101.42248904508));
#18652=CARTESIAN_POINT('Ctrl Pts',(178.577222120356,0.000324335621672112,
-101.429345386505));
#18653=CARTESIAN_POINT('Ctrl Pts',(178.574377192256,0.000405370262009153,
-101.437120258995));
#18654=CARTESIAN_POINT('Ctrl Pts',(178.571287400785,0.000508732071868225,
-101.445561210993));
#18655=CARTESIAN_POINT('Ctrl Pts',(178.568018800818,0.000639503791382112,
-101.454488825522));
#18656=CARTESIAN_POINT('Ctrl Pts',(178.562944383933,0.000842523502652618,
-101.468348716107));
#18657=CARTESIAN_POINT('Ctrl Pts',(178.557440800738,0.00111288774644858,
-101.483376639919));
#18658=CARTESIAN_POINT('Ctrl Pts',(178.551802736549,0.00145317996012051,
-101.498773356));
#18659=CARTESIAN_POINT('Ctrl Pts',(178.548206591168,0.0016702296833909,
-101.508593895026));
#18660=CARTESIAN_POINT('Ctrl Pts',(178.544556784656,0.00191520563125934,
-101.518561639214));
#18661=CARTESIAN_POINT('Ctrl Pts',(178.540921312626,0.00218441435491767,
-101.528492379834));
#18662=CARTESIAN_POINT('Ctrl Pts',(178.537513057598,0.00243679753334736,
-101.537802449165));
#18663=CARTESIAN_POINT('Ctrl Pts',(178.534117901125,0.00271033425977986,
-101.54707862243));
#18664=CARTESIAN_POINT('Ctrl Pts',(178.530774591244,0.00300072598369727,
-101.556216272597));
#18665=CARTESIAN_POINT('Ctrl Pts',(178.527853564307,0.00325443924329612,
-101.564199774942));
#18666=CARTESIAN_POINT('Ctrl Pts',(178.524972112737,0.00352092663549996,
-101.572077526154));
#18667=CARTESIAN_POINT('Ctrl Pts',(178.522139893218,0.00379788761149813,
-101.579824088899));
#18668=CARTESIAN_POINT('Ctrl Pts',(178.519478343991,0.00405815884639462,
-101.587103841739));
#18669=CARTESIAN_POINT('Ctrl Pts',(178.516860351853,0.00432761426520865,
-101.594267506857));
#18670=CARTESIAN_POINT('Ctrl Pts',(178.514277900784,0.00460593307088419,
-101.601338094426));
#18671=CARTESIAN_POINT('Ctrl Pts',(178.511799080951,0.00487308321503558,
-101.60812494623));
#18672=CARTESIAN_POINT('Ctrl Pts',(178.509353088197,0.0051483431981555,
-101.614825801238));
#18673=CARTESIAN_POINT('Ctrl Pts',(178.506916399187,0.00543380183925013,
-101.621506458109));
#18674=CARTESIAN_POINT('Ctrl Pts',(178.504429078999,0.00572519193357054,
-101.628325930199));
#18675=CARTESIAN_POINT('Ctrl Pts',(178.50194866006,0.00602751424299315,
-101.635132076566));
#18676=CARTESIAN_POINT('Ctrl Pts',(178.499444122459,0.00634483842667621,
-101.642011678311));
#18677=CARTESIAN_POINT('Ctrl Pts',(178.496859738753,0.00667227908863532,
-101.649110605734));
#18678=CARTESIAN_POINT('Ctrl Pts',(178.494249748556,0.0070157416033647,
-101.656287555538));
#18679=CARTESIAN_POINT('Ctrl Pts',(178.491600508035,0.00737805345699072,
-101.663581424513));
#18680=CARTESIAN_POINT('Ctrl Pts',(178.488804043098,0.00776049981719095,
-101.671280630633));
#18681=CARTESIAN_POINT('Ctrl Pts',(178.485963965907,0.00816399903704424,
-101.679109797114));
#18682=CARTESIAN_POINT('Ctrl Pts',(178.483084972836,0.00858931241530336,
-101.68705709765));
#18683=CARTESIAN_POINT('Ctrl Pts',(178.479986355456,0.00904707087224558,
-101.695610658898));
#18684=CARTESIAN_POINT('Ctrl Pts',(178.476842835217,0.00953016315957769,
-101.704300612999));
#18685=CARTESIAN_POINT('Ctrl Pts',(178.47368140586,0.0100356889235731,-101.713053049961));
#18686=CARTESIAN_POINT('Ctrl Pts',(178.470120265003,0.0106051302265015,
-101.722912090711));
#18687=CARTESIAN_POINT('Ctrl Pts',(178.466536704481,0.0112031337716295,
-101.732849644034));
#18688=CARTESIAN_POINT('Ctrl Pts',(178.462991613128,0.011819372271303,-101.742696590626));
#18689=CARTESIAN_POINT('Ctrl Pts',(178.456316716467,0.0129796606517407,
-101.761236973481));
#18690=CARTESIAN_POINT('Ctrl Pts',(178.449781177082,0.0142069873144255,
-101.779449700228));
#18691=CARTESIAN_POINT('Ctrl Pts',(178.443867730057,0.0153837152578814,
-101.795972224341));
#18692=CARTESIAN_POINT('Ctrl Pts',(178.440842416488,0.0159857280940882,
-101.804425131113));
#18693=CARTESIAN_POINT('Ctrl Pts',(178.437980334388,0.0165735927382017,
-101.812433997959));
#18694=CARTESIAN_POINT('Ctrl Pts',(178.435334953384,0.0171300092461038,
-101.819845063868));
#18695=CARTESIAN_POINT('Ctrl Pts',(178.432951108472,0.0176314155309591,
-101.826523433348));
#18696=CARTESIAN_POINT('Ctrl Pts',(178.430743438668,0.0181071457819583,
-101.832715725971));
#18697=CARTESIAN_POINT('Ctrl Pts',(178.428737030369,0.0185468694585307,
-101.838348235259));
#18698=CARTESIAN_POINT('Ctrl Pts',(178.426860560632,0.0189581158494036,
-101.843615973249));
#18699=CARTESIAN_POINT('Ctrl Pts',(178.425160261885,0.0193377870550568,
-101.848393671963));
#18700=CARTESIAN_POINT('Ctrl Pts',(178.423641411031,0.0196810600166027,
-101.852663957193));
#18701=CARTESIAN_POINT('Ctrl Pts',(178.422228645277,0.020000356860667,-101.856635981645));
#18702=CARTESIAN_POINT('Ctrl Pts',(178.420972900558,0.0202881342051908,
-101.860168883262));
#18703=CARTESIAN_POINT('Ctrl Pts',(178.419863717692,0.0205444722138255,
-101.863290454144));
#18704=CARTESIAN_POINT('Ctrl Pts',(178.418788174717,0.0207930358664343,
-101.866317352357));
#18705=CARTESIAN_POINT('Ctrl Pts',(178.417850536333,0.0210120087344738,
-101.868957207664));
#18706=CARTESIAN_POINT('Ctrl Pts',(178.417025849348,0.0212057651772088,
-101.871279308984));
#18707=CARTESIAN_POINT('Ctrl Pts',(178.416222831459,0.0213944305649158,
-101.87354039584));
#18708=CARTESIAN_POINT('Ctrl Pts',(178.415526991626,0.0215591700668775,
-101.875499968855));
#18709=CARTESIAN_POINT('Ctrl Pts',(178.414899116768,0.0217084973953576,
-101.877268125753));
#18710=CARTESIAN_POINT('Ctrl Pts',(178.414290865431,0.0218531576661837,
-101.878981020896));
#18711=CARTESIAN_POINT('Ctrl Pts',(178.41374644488,0.0219833464708782,-101.880514144137));
#18712=CARTESIAN_POINT('Ctrl Pts',(178.413213893231,0.0221112223987379,
-101.88201406864));
#18713=CARTESIAN_POINT('Ctrl Pts',(178.413125647366,0.0221324119336719,
-101.882262611921));
#18714=CARTESIAN_POINT('Ctrl Pts',(178.413037689107,0.0221535482572281,
-101.88251035271));
#18715=CARTESIAN_POINT('Ctrl Pts',(178.412949735578,0.0221746991903141,
-101.882758090243));
#18716=CARTESIAN_POINT('',(178.787524552389,0.000402961547082414,-102.019536869264));
#18717=CARTESIAN_POINT('Ctrl Pts',(178.787524552389,0.000402961547082414,
-102.019536869264));
#18718=CARTESIAN_POINT('Ctrl Pts',(178.662666280119,0.00766020742816023,
-101.973943942923));
#18719=CARTESIAN_POINT('Ctrl Pts',(178.537808007848,0.014917453309238,-101.928351016583));
#18720=CARTESIAN_POINT('Ctrl Pts',(178.412949735578,0.0221746991903159,
-101.882758090243));
#18721=CARTESIAN_POINT('',(178.812916258969,0.,-101.95));
#18722=CARTESIAN_POINT('Ctrl Pts',(178.787524552389,0.000402961547083081,
-102.019536869264));
#18723=CARTESIAN_POINT('Ctrl Pts',(178.78764841214,0.000399030350633984,
-102.019197688124));
#18724=CARTESIAN_POINT('Ctrl Pts',(178.787773880524,0.000395071002771159,
-102.01885410166));
#18725=CARTESIAN_POINT('Ctrl Pts',(178.78793361532,0.000390082847545159,
-102.018416679296));
#18726=CARTESIAN_POINT('Ctrl Pts',(178.788100783821,0.000384862554586033,
-102.017958900261));
#18727=CARTESIAN_POINT('Ctrl Pts',(178.788305342406,0.000378518970205901,
-102.01739873139));
#18728=CARTESIAN_POINT('Ctrl Pts',(178.788564734392,0.000370623383797231,
-102.016688404118));
#18729=CARTESIAN_POINT('Ctrl Pts',(178.788858149117,0.000361692185276813,
-102.015884907893));
#18730=CARTESIAN_POINT('Ctrl Pts',(178.789221715781,0.000350777275430554,
-102.014889304208));
#18731=CARTESIAN_POINT('Ctrl Pts',(178.789656465201,0.00033813726450127,
-102.013698766371));
#18732=CARTESIAN_POINT('Ctrl Pts',(178.790132138563,0.000324307420864918,
-102.012396160525));
#18733=CARTESIAN_POINT('Ctrl Pts',(178.790692580633,0.000308441360554114,
-102.010861415125));
#18734=CARTESIAN_POINT('Ctrl Pts',(178.791315549691,0.000291620850831009,
-102.009155432272));
#18735=CARTESIAN_POINT('Ctrl Pts',(178.792247224669,0.000266465110246515,
-102.006604067135));
#18736=CARTESIAN_POINT('Ctrl Pts',(178.793317070051,0.000239334836013709,
-102.003674304649));
#18737=CARTESIAN_POINT('Ctrl Pts',(178.794410700059,0.00021403709302259,
-102.000679377506));
#18738=CARTESIAN_POINT('Ctrl Pts',(178.795148224044,0.000196976759901188,
-101.998659653661));
#18739=CARTESIAN_POINT('Ctrl Pts',(178.795895454195,0.000180736351586767,
-101.9966133361));
#18740=CARTESIAN_POINT('Ctrl Pts',(178.796625704937,0.000165866021982986,
-101.994613504147));
#18741=CARTESIAN_POINT('Ctrl Pts',(178.797262035433,0.000152908220404063,
-101.992870877969));
#18742=CARTESIAN_POINT('Ctrl Pts',(178.797885231353,0.000140979679693556,
-101.991164211473));
#18743=CARTESIAN_POINT('Ctrl Pts',(178.798491417233,0.000130049363544771,
-101.989504119402));
#18744=CARTESIAN_POINT('Ctrl Pts',(178.799058386644,0.000119826171107409,
-101.987951424998));
#18745=CARTESIAN_POINT('Ctrl Pts',(178.799610286814,0.000110468349953339,
-101.986439991158));
#18746=CARTESIAN_POINT('Ctrl Pts',(178.800159818369,0.000101705604670599,
-101.984935038457));
#18747=CARTESIAN_POINT('Ctrl Pts',(178.800710252065,9.29284739725731E-5,
-101.983427615142));
#18748=CARTESIAN_POINT('Ctrl Pts',(178.801261406613,8.46980848399352E-5,
-101.981918212337));
#18749=CARTESIAN_POINT('Ctrl Pts',(178.801827369149,7.68530597206052E-5,
-101.980368253329));
#18750=CARTESIAN_POINT('Ctrl Pts',(178.802440098241,6.8359785321794E-5,
-101.978690218273));
#18751=CARTESIAN_POINT('Ctrl Pts',(178.803070001693,6.03342640516636E-5,
-101.976965145865));
#18752=CARTESIAN_POINT('Ctrl Pts',(178.803714099497,5.29252697356597E-5,
-101.975201199093));
#18753=CARTESIAN_POINT('Ctrl Pts',(178.804466950208,4.42653013113147E-5,
-101.973139418143));
#18754=CARTESIAN_POINT('Ctrl Pts',(178.805238896389,3.64757779670852E-5,
-101.971025339937));
#18755=CARTESIAN_POINT('Ctrl Pts',(178.806001069089,2.98874832731499E-5,
-101.968938028039));
#18756=CARTESIAN_POINT('Ctrl Pts',(178.806915993951,2.19787840815128E-5,
-101.96643238391));
#18757=CARTESIAN_POINT('Ctrl Pts',(178.807815215869,1.58466567429737E-5,
-101.963969744905));
#18758=CARTESIAN_POINT('Ctrl Pts',(178.808631227751,1.14758459881514E-5,
-101.961734991272));
#18759=CARTESIAN_POINT('Ctrl Pts',(178.809260196792,8.1068942553096E-6,
-101.960012478552));
#18760=CARTESIAN_POINT('Ctrl Pts',(178.809838942981,5.75949614264358E-6,
-101.958427509956));
#18761=CARTESIAN_POINT('Ctrl Pts',(178.810343455118,4.13699453183369E-6,
-101.957045843971));
#18762=CARTESIAN_POINT('Ctrl Pts',(178.810801738817,2.66316271661563E-6,
-101.955790780017));
#18763=CARTESIAN_POINT('Ctrl Pts',(178.811198450184,1.77620580733071E-6,
-101.95470434237));
#18764=CARTESIAN_POINT('Ctrl Pts',(178.811528375133,1.20384667301465E-6,
-101.953800810259));
#18765=CARTESIAN_POINT('Ctrl Pts',(178.811837957088,6.66778893284302E-7,
-101.95295298945));
#18766=CARTESIAN_POINT('Ctrl Pts',(178.812088533466,4.02530379490208E-7,
-101.952266765043));
#18767=CARTESIAN_POINT('Ctrl Pts',(178.812291139739,2.44220887957169E-7,
-101.951711914309));
#18768=CARTESIAN_POINT('Ctrl Pts',(178.812480730277,9.60814393472537E-8,
-101.951192708032));
#18769=CARTESIAN_POINT('Ctrl Pts',(178.812628230417,4.12488927176395E-8,
-101.950788772916));
#18770=CARTESIAN_POINT('Ctrl Pts',(178.812758452829,1.55631960652158E-8,
-101.950432155475));
#18771=CARTESIAN_POINT('Ctrl Pts',(178.812812952405,4.81343668080793E-9,
-101.950282906975));
#18772=CARTESIAN_POINT('Ctrl Pts',(178.812864631041,0.,-101.950141384054));
#18773=CARTESIAN_POINT('Ctrl Pts',(178.812916258969,0.,-101.95));
#18774=CARTESIAN_POINT('',(178.706458129484,2.77555756156289E-16,-101.658452405258));
#18775=CARTESIAN_POINT('Ctrl Pts',(178.787524039848,5.93046172723724,-107.949597022186));
#18776=CARTESIAN_POINT('Ctrl Pts',(178.788055468328,5.9319170065127,-107.949613889587));
#18777=CARTESIAN_POINT('Ctrl Pts',(178.789730276056,5.93650327150383,-107.94967251859));
#18778=CARTESIAN_POINT('Ctrl Pts',(178.796663949731,5.95549109773913,-107.949843338737));
#18779=CARTESIAN_POINT('Ctrl Pts',(178.802274889545,5.9708572965487,-107.949940304033));
#18780=CARTESIAN_POINT('Ctrl Pts',(178.808321541956,5.98741690531324,-107.949992199559));
#18781=CARTESIAN_POINT('Ctrl Pts',(178.811886383268,5.99717964379856,-107.950000306293));
#18782=CARTESIAN_POINT('Ctrl Pts',(178.812561951533,5.99902972241609,-107.95));
#18783=CARTESIAN_POINT('Ctrl Pts',(178.812916258969,6.,-107.95));
#18784=CARTESIAN_POINT('Ctrl Pts',(178.662665771413,5.97605465101009,-107.942339741564));
#18785=CARTESIAN_POINT('Ctrl Pts',(178.664312652826,5.98062783599467,-107.942427298381));
#18786=CARTESIAN_POINT('Ctrl Pts',(178.670769881366,5.99845250694587,-107.943108688047));
#18787=CARTESIAN_POINT('Ctrl Pts',(178.689813167772,6.05087787990199,-107.94503083354));
#18788=CARTESIAN_POINT('Ctrl Pts',(178.70976624133,6.1058117496159,-107.947239781462));
#18789=CARTESIAN_POINT('Ctrl Pts',(178.727201696273,6.15378129306144,-107.948897276685));
#18790=CARTESIAN_POINT('Ctrl Pts',(178.737862493431,6.18311815560049,-107.949788255786));
#18791=CARTESIAN_POINT('Ctrl Pts',(178.740836000836,6.19131037031829,-107.95));
#18792=CARTESIAN_POINT('Ctrl Pts',(178.741944172646,6.1943650631615,-107.95));
#18793=CARTESIAN_POINT('Ctrl Pts',(178.537807502978,6.02164757478294,-107.935082460943));
#18794=CARTESIAN_POINT('Ctrl Pts',(178.540562604801,6.02935581973102,-107.935472908878));
#18795=CARTESIAN_POINT('Ctrl Pts',(178.548140009852,6.05016876508724,-107.93751448423));
#18796=CARTESIAN_POINT('Ctrl Pts',(178.587637169058,6.15753734426006,-107.942617344146));
#18797=CARTESIAN_POINT('Ctrl Pts',(178.614548799958,6.23191679011827,-107.946864743799));
#18798=CARTESIAN_POINT('Ctrl Pts',(178.64762791374,6.32331090469419,-107.948970766507));
#18799=CARTESIAN_POINT('Ctrl Pts',(178.666539875963,6.37617477796488,-107.949592686699));
#18800=CARTESIAN_POINT('Ctrl Pts',(178.669110050139,6.3835910182205,-107.95));
#18801=CARTESIAN_POINT('Ctrl Pts',(178.670972086323,6.38873012632301,-107.95));
#18802=CARTESIAN_POINT('Ctrl Pts',(178.412949234542,6.06724049855578,-107.927825180321));
#18803=CARTESIAN_POINT('Ctrl Pts',(178.416788814167,6.07805539364222,-107.9287485193));
#18804=CARTESIAN_POINT('Ctrl Pts',(178.428797505081,6.11209602694949,-107.931943728692));
#18805=CARTESIAN_POINT('Ctrl Pts',(178.47931211943,6.25289954945229,-107.941313577143));
#18806=CARTESIAN_POINT('Ctrl Pts',(178.520871373432,6.36685401704756,-107.946698106754));
#18807=CARTESIAN_POINT('Ctrl Pts',(178.565883366218,6.48966771290196,-107.94957040054));
#18808=CARTESIAN_POINT('Ctrl Pts',(178.592383761069,6.56211168242985,-107.950016726301));
#18809=CARTESIAN_POINT('Ctrl Pts',(178.597384099442,6.57587166612271,-107.95));
#18810=CARTESIAN_POINT('Ctrl Pts',(178.6,6.58309518948451,-107.95));
#18811=CARTESIAN_POINT('',(178.812916258969,6.,-107.95));
#18812=CARTESIAN_POINT('',(178.787524039848,5.93046172723724,-107.949597022186));
#18813=CARTESIAN_POINT('Ctrl Pts',(178.812916258969,6.,-107.95));
#18814=CARTESIAN_POINT('Ctrl Pts',(178.8127923898,5.99966078194887,-107.95));
#18815=CARTESIAN_POINT('Ctrl Pts',(178.812666912034,5.99931715853558,-107.949999977092));
#18816=CARTESIAN_POINT('Ctrl Pts',(178.812507168478,5.99887969296171,-107.949999895409));
#18817=CARTESIAN_POINT('Ctrl Pts',(178.812339990794,5.99842186866603,-107.949999809925));
#18818=CARTESIAN_POINT('Ctrl Pts',(178.812135423695,5.99786164766841,-107.949999661008));
#18819=CARTESIAN_POINT('Ctrl Pts',(178.811876024087,5.99715125904428,-107.949999323723));
#18820=CARTESIAN_POINT('Ctrl Pts',(178.811582600943,5.99634769397784,-107.949998942198));
#18821=CARTESIAN_POINT('Ctrl Pts',(178.811219027098,5.99535200993297,-107.949998317815));
#18822=CARTESIAN_POINT('Ctrl Pts',(178.810784271547,5.99416138284707,-107.949997159212));
#18823=CARTESIAN_POINT('Ctrl Pts',(178.810308592617,5.99285868247457,-107.94999589155));
#18824=CARTESIAN_POINT('Ctrl Pts',(178.809748146635,5.99132383326824,-107.94999396957));
#18825=CARTESIAN_POINT('Ctrl Pts',(178.809125174401,5.98961774499851,-107.949991017392));
#18826=CARTESIAN_POINT('Ctrl Pts',(178.808193484888,5.98706619540862,-107.949986602245));
#18827=CARTESIAN_POINT('Ctrl Pts',(178.807123623593,5.98413623812711,-107.949979775947));
#18828=CARTESIAN_POINT('Ctrl Pts',(178.806029976263,5.98114113876119,-107.949970361873));
#18829=CARTESIAN_POINT('Ctrl Pts',(178.805292443291,5.97912130615377,-107.949964013218));
#18830=CARTESIAN_POINT('Ctrl Pts',(178.8045452036,5.9770748900843,-107.949956536432));
#18831=CARTESIAN_POINT('Ctrl Pts',(178.803814942577,5.97507497391497,-107.949948228366));
#18832=CARTESIAN_POINT('Ctrl Pts',(178.803178603945,5.97333227660838,-107.949940988841));
#18833=CARTESIAN_POINT('Ctrl Pts',(178.802555399287,5.97162554958125,-107.949933136853));
#18834=CARTESIAN_POINT('Ctrl Pts',(178.801949204102,5.96996540809482,-107.94992482647));
#18835=CARTESIAN_POINT('Ctrl Pts',(178.801382229386,5.96841267678133,-107.949917053764));
#18836=CARTESIAN_POINT('Ctrl Pts',(178.800830323213,5.96690121509211,-107.949908893929));
#18837=CARTESIAN_POINT('Ctrl Pts',(178.800280785516,5.96539624482733,-107.949900214181));
#18838=CARTESIAN_POINT('Ctrl Pts',(178.799730342856,5.96388879622168,-107.949891520139));
#18839=CARTESIAN_POINT('Ctrl Pts',(178.799179179282,5.96237937864897,-107.949882256457));
#18840=CARTESIAN_POINT('Ctrl Pts',(178.798613206928,5.96082941367589,-107.949872137401));
#18841=CARTESIAN_POINT('Ctrl Pts',(178.798000470593,5.95915138143477,-107.94986118225));
#18842=CARTESIAN_POINT('Ctrl Pts',(178.797370559173,5.95742632285293,-107.949849214239));
#18843=CARTESIAN_POINT('Ctrl Pts',(178.796726452316,5.95566239958307,-107.949836179196));
#18844=CARTESIAN_POINT('Ctrl Pts',(178.795973597401,5.9536006635722,-107.949820943375));
#18845=CARTESIAN_POINT('Ctrl Pts',(178.795201645861,5.95148664466333,-107.949804231078));
#18846=CARTESIAN_POINT('Ctrl Pts',(178.794439465761,5.94939939913607,-107.949786627805));
#18847=CARTESIAN_POINT('Ctrl Pts',(178.793524504241,5.94689375861677,-107.949765495901));
#18848=CARTESIAN_POINT('Ctrl Pts',(178.79262524356,5.944431135813,-107.949743085817));
#18849=CARTESIAN_POINT('Ctrl Pts',(178.791809196363,5.94219640766138,-107.949721555598));
#18850=CARTESIAN_POINT('Ctrl Pts',(178.791180207509,5.94047393486153,-107.949704960642));
#18851=CARTESIAN_POINT('Ctrl Pts',(178.790601442454,5.9388890082226,-107.949688938252));
#18852=CARTESIAN_POINT('Ctrl Pts',(178.790096914054,5.93750738102304,-107.949674547221));
#18853=CARTESIAN_POINT('Ctrl Pts',(178.789638616417,5.93625235458416,-107.949661474864));
#18854=CARTESIAN_POINT('Ctrl Pts',(178.789241893049,5.93516595105505,-107.949649769988));
#18855=CARTESIAN_POINT('Ctrl Pts',(178.788911959032,5.93426244786692,-107.949639870379));
#18856=CARTESIAN_POINT('Ctrl Pts',(178.788602368806,5.93341465484948,-107.949630581182));
#18857=CARTESIAN_POINT('Ctrl Pts',(178.788351786654,5.93272845333488,-107.949622892056));
#18858=CARTESIAN_POINT('Ctrl Pts',(178.788149177667,5.93217362299574,-107.949616619633));
#18859=CARTESIAN_POINT('Ctrl Pts',(178.787959584857,5.9316544365331,-107.949610750169));
#18860=CARTESIAN_POINT('Ctrl Pts',(178.787812085006,5.93125051870808,-107.949606123405));
#18861=CARTESIAN_POINT('Ctrl Pts',(178.787681865722,5.93089392231775,-107.94960201597));
#18862=CARTESIAN_POINT('Ctrl Pts',(178.787627358605,5.93074465839335,-107.949600296682));
#18863=CARTESIAN_POINT('Ctrl Pts',(178.787575673856,5.9306031233133,-107.949598661036));
#18864=CARTESIAN_POINT('Ctrl Pts',(178.787524039848,5.93046172723724,-107.949597022186));
#18865=CARTESIAN_POINT('',(178.412949234542,6.06724049855578,-107.927825180321));
#18866=CARTESIAN_POINT('Ctrl Pts',(178.412949234542,6.06724049855578,-107.927825180321));
#18867=CARTESIAN_POINT('Ctrl Pts',(178.537807502978,6.02164757478294,-107.935082460943));
#18868=CARTESIAN_POINT('Ctrl Pts',(178.662665771413,5.97605465101009,-107.942339741564));
#18869=CARTESIAN_POINT('Ctrl Pts',(178.787524039848,5.93046172723724,-107.949597022186));
#18870=CARTESIAN_POINT('',(178.6,6.58309518948451,-107.95));
#18871=CARTESIAN_POINT('Ctrl Pts',(178.412949234542,6.06724049855578,-107.927825180321));
#18872=CARTESIAN_POINT('Ctrl Pts',(178.413479203313,6.06873325484981,-107.927952626779));
#18873=CARTESIAN_POINT('Ctrl Pts',(178.414010755826,6.07023015200046,-107.928079922666));
#18874=CARTESIAN_POINT('Ctrl Pts',(178.414598463368,6.07188520349623,-107.928219936917));
#18875=CARTESIAN_POINT('Ctrl Pts',(178.415213505117,6.07361723123663,-107.928366463213));
#18876=CARTESIAN_POINT('Ctrl Pts',(178.415890038074,6.07552244369575,-107.928526920857));
#18877=CARTESIAN_POINT('Ctrl Pts',(178.416671529666,6.07772300303662,-107.928710903972));
#18878=CARTESIAN_POINT('Ctrl Pts',(178.417481884439,6.0800048366274,-107.928901682219));
#18879=CARTESIAN_POINT('Ctrl Pts',(178.418405026846,6.08260404766235,-107.929117745108));
#18880=CARTESIAN_POINT('Ctrl Pts',(178.419469997538,6.08560145625783,-107.929364432221));
#18881=CARTESIAN_POINT('Ctrl Pts',(178.420583048303,6.0887341884148,-107.92962225648));
#18882=CARTESIAN_POINT('Ctrl Pts',(178.421850942572,6.09230165151869,-107.929913509125));
#18883=CARTESIAN_POINT('Ctrl Pts',(178.423287109935,6.09633987574133,-107.930238780429));
#18884=CARTESIAN_POINT('Ctrl Pts',(178.424806597946,6.10061238147632,-107.930582922664));
#18885=CARTESIAN_POINT('Ctrl Pts',(178.426514350532,6.10541155145395,-107.930965095528));
#18886=CARTESIAN_POINT('Ctrl Pts',(178.428406024718,6.11072251269353,-107.931380513992));
#18887=CARTESIAN_POINT('Ctrl Pts',(178.430450932505,6.11646368422914,-107.931829583108));
#18888=CARTESIAN_POINT('Ctrl Pts',(178.43271062602,6.12280247841158,-107.932317405234));
#18889=CARTESIAN_POINT('Ctrl Pts',(178.435158382966,6.1296602790685,-107.932832831001));
#18890=CARTESIAN_POINT('Ctrl Pts',(178.437934870285,6.13743907287411,-107.933417477737));
#18891=CARTESIAN_POINT('Ctrl Pts',(178.440953077155,6.14588483863718,-107.93403743716));
#18892=CARTESIAN_POINT('Ctrl Pts',(178.444150457434,6.15481772739735,-107.934672492242));
#18893=CARTESIAN_POINT('Ctrl Pts',(178.449103370998,6.16865525126056,-107.93565622663));
#18894=CARTESIAN_POINT('Ctrl Pts',(178.454484757555,6.18365673275744,-107.936674546861));
#18895=CARTESIAN_POINT('Ctrl Pts',(178.460013146549,6.19902659477107,-107.937657083293));
#18896=CARTESIAN_POINT('Ctrl Pts',(178.463544791462,6.20884516850738,-107.938284747119));
#18897=CARTESIAN_POINT('Ctrl Pts',(178.467135303381,6.21881124737588,-107.938898064687));
#18898=CARTESIAN_POINT('Ctrl Pts',(178.47071856603,6.2287406065041,-107.939484838886));
#18899=CARTESIAN_POINT('Ctrl Pts',(178.474077874763,6.23804938068681,-107.940034939697));
#18900=CARTESIAN_POINT('Ctrl Pts',(178.477430296671,6.24732450793906,-107.940561734482));
#18901=CARTESIAN_POINT('Ctrl Pts',(178.480737796232,6.25646134033518,-107.94106038123));
#18902=CARTESIAN_POINT('Ctrl Pts',(178.483628027253,6.26444548543807,-107.94149611955));
#18903=CARTESIAN_POINT('Ctrl Pts',(178.486483935739,6.27232401612018,-107.94191045257));
#18904=CARTESIAN_POINT('Ctrl Pts',(178.489295938703,6.28007146975104,-107.94230335782));
#18905=CARTESIAN_POINT('Ctrl Pts',(178.49193892756,6.28735326634753,-107.942672647685));
#18906=CARTESIAN_POINT('Ctrl Pts',(178.49454303769,6.29451903346483,-107.943023052383));
#18907=CARTESIAN_POINT('Ctrl Pts',(178.497116199141,6.30159180694569,-107.94335674417));
#18908=CARTESIAN_POINT('Ctrl Pts',(178.499585573981,6.30837930520869,-107.943676976741));
#18909=CARTESIAN_POINT('Ctrl Pts',(178.502026355481,6.31508092194477,-107.94398185317));
#18910=CARTESIAN_POINT('Ctrl Pts',(178.504461997836,6.32176249687495,-107.944274820287));
#18911=CARTESIAN_POINT('Ctrl Pts',(178.506947342092,6.32858041652259,-107.944573765714));
#18912=CARTESIAN_POINT('Ctrl Pts',(178.509430123365,6.33538518866083,-107.944860667827));
#18913=CARTESIAN_POINT('Ctrl Pts',(178.511941391018,6.34226352759025,-107.94513878121));
#18914=CARTESIAN_POINT('Ctrl Pts',(178.514532849449,6.34936150832142,-107.945425775418));
#18915=CARTESIAN_POINT('Ctrl Pts',(178.51715458036,6.35653763787409,-107.94570334598));
#18916=CARTESIAN_POINT('Ctrl Pts',(178.519820335973,6.36383079184547,-107.94597187229));
#18917=CARTESIAN_POINT('Ctrl Pts',(178.522634229987,6.37152923284386,-107.946255320844));
#18918=CARTESIAN_POINT('Ctrl Pts',(178.525497070125,6.37935775149736,-107.946528613934));
#18919=CARTESIAN_POINT('Ctrl Pts',(178.528404154866,6.3873045340961,-107.946789831109));
#18920=CARTESIAN_POINT('Ctrl Pts',(178.531532994176,6.39585750313594,-107.947070974124));
#18921=CARTESIAN_POINT('Ctrl Pts',(178.53471292725,6.40454701494677,-107.947338023315));
#18922=CARTESIAN_POINT('Ctrl Pts',(178.537916535956,6.41329921114082,-107.947587389251));
#18923=CARTESIAN_POINT('Ctrl Pts',(178.541525048346,6.42315759626256,-107.947868272515));
#18924=CARTESIAN_POINT('Ctrl Pts',(178.545163323259,6.43309474441174,-107.948126551975));
#18925=CARTESIAN_POINT('Ctrl Pts',(178.54876895076,6.44294166046983,-107.948357926994));
#18926=CARTESIAN_POINT('Ctrl Pts',(178.555559818195,6.46148742028091,-107.948793700539));
#18927=CARTESIAN_POINT('Ctrl Pts',(178.562232479394,6.47970668810108,-107.949130963775));
#18928=CARTESIAN_POINT('Ctrl Pts',(178.56828435694,6.49623651029247,-107.949371076525));
#18929=CARTESIAN_POINT('Ctrl Pts',(178.571379491104,6.50469041852403,-107.949493878279));
#18930=CARTESIAN_POINT('Ctrl Pts',(178.5743116503,6.51270076910019,-107.949592066599));
#18931=CARTESIAN_POINT('Ctrl Pts',(178.577024251211,6.52011387104887,-107.949670003794));
#18932=CARTESIAN_POINT('Ctrl Pts',(178.579468755426,6.52679430784969,-107.949740238159));
#18933=CARTESIAN_POINT('Ctrl Pts',(178.581734724378,6.53298908286734,-107.949794115064));
#18934=CARTESIAN_POINT('Ctrl Pts',(178.583795074241,6.53862447881607,-107.949835858399));
#18935=CARTESIAN_POINT('Ctrl Pts',(178.585722016495,6.54389498299908,-107.949874898855));
#18936=CARTESIAN_POINT('Ctrl Pts',(178.587468955848,6.54867578942129,-107.949903374666));
#18937=CARTESIAN_POINT('Ctrl Pts',(178.589029536264,6.55294946252688,-107.949924777042));
#18938=CARTESIAN_POINT('Ctrl Pts',(178.590481114101,6.55692463041785,-107.949944684516));
#18939=CARTESIAN_POINT('Ctrl Pts',(178.591771416975,6.56046091966274,-107.949958491691));
#18940=CARTESIAN_POINT('Ctrl Pts',(178.592910673727,6.5635860256236,-107.949968587791));
#18941=CARTESIAN_POINT('Ctrl Pts',(178.594015383929,6.56661636661492,-107.94997837774));
#18942=CARTESIAN_POINT('Ctrl Pts',(178.594977967003,6.56925979976113,-107.949984684072));
#18943=CARTESIAN_POINT('Ctrl Pts',(178.595823866001,6.57158547788136,-107.949989099866));
#18944=CARTESIAN_POINT('Ctrl Pts',(178.596647541579,6.57385005588911,-107.949993399649));
#18945=CARTESIAN_POINT('Ctrl Pts',(178.597360497027,6.57581311704121,-107.949995903734));
#18946=CARTESIAN_POINT('Ctrl Pts',(178.598003120442,6.57758458484291,-107.949997507791));
#18947=CARTESIAN_POINT('Ctrl Pts',(178.598625651554,6.57930066582568,-107.949999061696));
#18948=CARTESIAN_POINT('Ctrl Pts',(178.599182131485,6.5808368133178,-107.949999767001));
#18949=CARTESIAN_POINT('Ctrl Pts',(178.599726292418,6.58233938722526,-107.949999953178));
#18950=CARTESIAN_POINT('Ctrl Pts',(178.599817733258,6.58259187984708,-107.949999984463));
#18951=CARTESIAN_POINT('Ctrl Pts',(178.599908867259,6.58284353638597,-107.95));
#18952=CARTESIAN_POINT('Ctrl Pts',(178.6,6.58309518948451,-107.95));
#18953=CARTESIAN_POINT('',(178.706458129484,6.29154759474225,-107.95));
#18954=CARTESIAN_POINT('Ctrl Pts',(178.412949234542,6.06724049855578,-107.927825180321));
#18955=CARTESIAN_POINT('Ctrl Pts',(178.240471965366,5.58142596856032,-107.886347987194));
#18956=CARTESIAN_POINT('Ctrl Pts',(178.066773026242,5.05523969179933,-107.780573504214));
#18957=CARTESIAN_POINT('Ctrl Pts',(177.858376158784,4.15716129915578,-107.487588730723));
#18958=CARTESIAN_POINT('Ctrl Pts',(177.799999999912,3.77824139277387,-107.327421746315));
#18959=CARTESIAN_POINT('Ctrl Pts',(177.8,3.42868316199151,-107.149999999604));
#18960=CARTESIAN_POINT('Ctrl Pts',(178.537807502978,6.02164757478294,-107.935082460943));
#18961=CARTESIAN_POINT('Ctrl Pts',(178.363767312538,5.53583597592066,-107.905551798508));
#18962=CARTESIAN_POINT('Ctrl Pts',(178.183613995588,5.01057297796046,-107.812220700977));
#18963=CARTESIAN_POINT('Ctrl Pts',(177.955395688911,4.11610793281407,-107.53590212866));
#18964=CARTESIAN_POINT('Ctrl Pts',(177.885823288832,3.73937765491853,-107.381196742299));
#18965=CARTESIAN_POINT('Ctrl Pts',(177.872973082299,3.39266652940119,-107.206172926527));
#18966=CARTESIAN_POINT('Ctrl Pts',(178.662665771413,5.97605465101009,-107.942339741564));
#18967=CARTESIAN_POINT('Ctrl Pts',(178.486832509378,5.49026482889952,-107.924762702489));
#18968=CARTESIAN_POINT('Ctrl Pts',(178.300397762631,4.96591073123605,-107.843861291125));
#18969=CARTESIAN_POINT('Ctrl Pts',(178.052417412725,4.07505247364037,-107.58421556635));
#18970=CARTESIAN_POINT('Ctrl Pts',(177.971553851954,3.70051482129146,-107.434941903923));
#18971=CARTESIAN_POINT('Ctrl Pts',(177.945946164598,3.35664989681088,-107.262345853449));
#18972=CARTESIAN_POINT('Ctrl Pts',(178.787524039848,5.93046172723724,-107.949597022186));
#18973=CARTESIAN_POINT('Ctrl Pts',(178.61012785655,5.44467483625986,-107.943966513803));
#18974=CARTESIAN_POINT('Ctrl Pts',(178.417238731978,4.92124401739719,-107.875508487888));
#18975=CARTESIAN_POINT('Ctrl Pts',(178.149436942852,4.03399910729865,-107.632528964287));
#18976=CARTESIAN_POINT('Ctrl Pts',(178.057377140874,3.66165108343612,-107.488716899907));
#18977=CARTESIAN_POINT('Ctrl Pts',(178.018919246896,3.32063326422056,-107.318518780371));
#18978=CARTESIAN_POINT('',(178.018919246896,3.32063326422068,-107.318518780371));
#18979=CARTESIAN_POINT('Ctrl Pts',(178.787524039848,5.93046172723724,-107.949597022186));
#18980=CARTESIAN_POINT('Ctrl Pts',(178.61012785655,5.44467483625986,-107.943966513803));
#18981=CARTESIAN_POINT('Ctrl Pts',(178.417238731978,4.92124401739719,-107.875508487888));
#18982=CARTESIAN_POINT('Ctrl Pts',(178.149436942852,4.03399910729865,-107.632528964287));
#18983=CARTESIAN_POINT('Ctrl Pts',(178.057377140874,3.66165108343612,-107.488716899907));
#18984=CARTESIAN_POINT('Ctrl Pts',(178.018919246896,3.32063326422056,-107.318518780371));
#18985=CARTESIAN_POINT('',(177.8,3.42868316190266,-107.14999999978));
#18986=CARTESIAN_POINT('',(178.018919246896,3.32063326422068,-107.318518780371));
#18987=CARTESIAN_POINT('Ctrl Pts',(177.8,3.42868316199151,-107.149999999604));
#18988=CARTESIAN_POINT('Ctrl Pts',(177.799999999912,3.77824139277387,-107.327421746315));
#18989=CARTESIAN_POINT('Ctrl Pts',(177.858376158784,4.15716129915578,-107.487588730723));
#18990=CARTESIAN_POINT('Ctrl Pts',(178.066773026242,5.05523969179933,-107.780573504214));
#18991=CARTESIAN_POINT('Ctrl Pts',(178.240471965366,5.58142596856032,-107.886347987194));
#18992=CARTESIAN_POINT('Ctrl Pts',(178.412949234542,6.06724049855578,-107.927825180321));
#18993=CARTESIAN_POINT('Origin',(177.9,6.00000000000001,-101.95));
#18994=CARTESIAN_POINT('',(177.8,3.10645162089483,-106.976666666667));
#18995=CARTESIAN_POINT('',(178.,3.00667409058086,-107.15));
#18996=CARTESIAN_POINT('',(177.8,3.10645162089483,-106.976666666667));
#18997=CARTESIAN_POINT('',(178.,0.800000000000001,-104.943325909419));
#18998=CARTESIAN_POINT('Origin',(178.,6.00000000000001,-101.95));
#18999=CARTESIAN_POINT('',(177.8,0.97333333333333,-104.843548379105));
#19000=CARTESIAN_POINT('',(178.,0.800000000000001,-104.943325909419));
#19001=CARTESIAN_POINT('Origin',(177.8,6.00000000000001,-101.95));
#19002=CARTESIAN_POINT('Ctrl Pts',(177.8,3.42868316199162,-107.149999999604));
#19003=CARTESIAN_POINT('Ctrl Pts',(177.8,3.31801931336447,-107.093831465749));
#19004=CARTESIAN_POINT('Ctrl Pts',(177.8,3.21069598181731,-107.036673848678));
#19005=CARTESIAN_POINT('Ctrl Pts',(177.8,3.10645162089484,-106.976666666667));
#19006=CARTESIAN_POINT('Ctrl Pts',(177.872973082299,3.39266652940131,-107.206172926527));
#19007=CARTESIAN_POINT('Ctrl Pts',(177.868914723125,3.28290392767113,-107.150766682816));
#19008=CARTESIAN_POINT('Ctrl Pts',(177.866666666667,3.17639835547358,-107.093853853762));
#19009=CARTESIAN_POINT('Ctrl Pts',(177.866666666667,3.07319244412352,-107.034444444444));
#19010=CARTESIAN_POINT('Ctrl Pts',(177.945946164598,3.35664989681099,-107.262345853449));
#19011=CARTESIAN_POINT('Ctrl Pts',(177.937829446251,3.24778854197779,-107.207701899883));
#19012=CARTESIAN_POINT('Ctrl Pts',(177.933333333333,3.14210072912985,-107.151033858845));
#19013=CARTESIAN_POINT('Ctrl Pts',(177.933333333333,3.0399332673522,-107.092222222222));
#19014=CARTESIAN_POINT('Ctrl Pts',(178.018919246896,3.32063326422067,-107.318518780371));
#19015=CARTESIAN_POINT('Ctrl Pts',(178.006744169376,3.21267315628445,-107.26463711695));
#19016=CARTESIAN_POINT('Ctrl Pts',(178.,3.10780310278612,-107.208213863928));
#19017=CARTESIAN_POINT('Ctrl Pts',(178.,3.00667409058087,-107.15));
#19018=CARTESIAN_POINT('Ctrl Pts',(177.8,3.10645162089484,-106.976666666667));
#19019=CARTESIAN_POINT('Ctrl Pts',(177.8,3.21069598181731,-107.036673848678));
#19020=CARTESIAN_POINT('Ctrl Pts',(177.8,3.31801931336447,-107.093831465749));
#19021=CARTESIAN_POINT('Ctrl Pts',(177.8,3.42868316199162,-107.149999999604));
#19022=CARTESIAN_POINT('Ctrl Pts',(178.018919246896,3.32063326422067,-107.318518780371));
#19023=CARTESIAN_POINT('Ctrl Pts',(178.006744169376,3.21267315628445,-107.26463711695));
#19024=CARTESIAN_POINT('Ctrl Pts',(178.,3.10780310278612,-107.208213863928));
#19025=CARTESIAN_POINT('Ctrl Pts',(178.,3.00667409058087,-107.15));
#19026=CARTESIAN_POINT('Ctrl Pts',(177.8,0.800000000395799,-104.521316838008));
#19027=CARTESIAN_POINT('Ctrl Pts',(177.799999999912,0.622578253685065,-104.171758607226));
#19028=CARTESIAN_POINT('Ctrl Pts',(177.858375951321,0.462411299210277,-103.79283930267));
#19029=CARTESIAN_POINT('Ctrl Pts',(178.066773083588,0.169426307367239,-102.894760003766));
#19030=CARTESIAN_POINT('Ctrl Pts',(178.240470897403,0.0636521521020384,
-102.368576933864));
#19031=CARTESIAN_POINT('Ctrl Pts',(178.412949735578,0.0221746991903157,
-101.882758090243));
#19032=CARTESIAN_POINT('Ctrl Pts',(177.872973082299,0.743827073473454,-104.557333470599));
#19033=CARTESIAN_POINT('Ctrl Pts',(177.885823288774,0.568803257717161,-104.210622345397));
#19034=CARTESIAN_POINT('Ctrl Pts',(177.955395481534,0.414097901249308,-103.83389266854));
#19035=CARTESIAN_POINT('Ctrl Pts',(178.183614063642,0.137779119795014,-102.939426720499));
#19036=CARTESIAN_POINT('Ctrl Pts',(178.363766257608,0.0444483646880333,
-102.414166925692));
#19037=CARTESIAN_POINT('Ctrl Pts',(178.537808007848,0.014917453309238,-101.928351016583));
#19038=CARTESIAN_POINT('Ctrl Pts',(177.945946164598,0.687654146551109,-104.593350103189));
#19039=CARTESIAN_POINT('Ctrl Pts',(177.971553852012,0.515058096060438,-104.249485178393));
#19040=CARTESIAN_POINT('Ctrl Pts',(178.052417640032,0.36578440471743,-103.874946934064));
#19041=CARTESIAN_POINT('Ctrl Pts',(178.300397980669,0.106138520890286,-102.984088610155));
#19042=CARTESIAN_POINT('Ctrl Pts',(178.486834293191,0.0252371025851526,
-102.4597302221));
#19043=CARTESIAN_POINT('Ctrl Pts',(178.662666280119,0.00766020742816018,
-101.973943942923));
#19044=CARTESIAN_POINT('Ctrl Pts',(178.018919246896,0.631481219628764,-104.629366735779));
#19045=CARTESIAN_POINT('Ctrl Pts',(178.057377140874,0.461283100092534,-104.288348916564));
#19046=CARTESIAN_POINT('Ctrl Pts',(178.149437170246,0.317471006756462,-103.916000299934));
#19047=CARTESIAN_POINT('Ctrl Pts',(178.417238960723,0.0744913333180605,
-103.028755326887));
#19048=CARTESIAN_POINT('Ctrl Pts',(178.610129653397,0.0060333151711475,
-102.505320213928));
#19049=CARTESIAN_POINT('Ctrl Pts',(178.787524552389,0.000402961547082414,
-102.019536869264));
#19050=CARTESIAN_POINT('',(177.8,0.800000000220451,-104.521316838097));
#19051=CARTESIAN_POINT('Ctrl Pts',(178.412949735578,0.0221746991903157,
-101.882758090243));
#19052=CARTESIAN_POINT('Ctrl Pts',(178.240470897403,0.0636521521020384,
-102.368576933864));
#19053=CARTESIAN_POINT('Ctrl Pts',(178.066773083588,0.169426307367239,-102.894760003766));
#19054=CARTESIAN_POINT('Ctrl Pts',(177.858375951321,0.462411299210277,-103.79283930267));
#19055=CARTESIAN_POINT('Ctrl Pts',(177.799999999912,0.622578253685065,-104.171758607226));
#19056=CARTESIAN_POINT('Ctrl Pts',(177.8,0.800000000395799,-104.521316838008));
#19057=CARTESIAN_POINT('',(178.018919246896,0.631481219628702,-104.629366735779));
#19058=CARTESIAN_POINT('',(177.8,0.800000000220451,-104.521316838097));
#19059=CARTESIAN_POINT('Ctrl Pts',(178.018919246896,0.631481219628764,-104.629366735779));
#19060=CARTESIAN_POINT('Ctrl Pts',(178.057377140874,0.461283100092534,-104.288348916564));
#19061=CARTESIAN_POINT('Ctrl Pts',(178.149437170246,0.317471006756462,-103.916000299934));
#19062=CARTESIAN_POINT('Ctrl Pts',(178.417238960723,0.0744913333180605,
-103.028755326887));
#19063=CARTESIAN_POINT('Ctrl Pts',(178.610129653397,0.0060333151711475,
-102.505320213928));
#19064=CARTESIAN_POINT('Ctrl Pts',(178.787524552389,0.000402961547082414,
-102.019536869264));
#19065=CARTESIAN_POINT('Ctrl Pts',(177.8,0.973333333333337,-104.843548379105));
#19066=CARTESIAN_POINT('Ctrl Pts',(177.8,0.913326151321774,-104.739304018183));
#19067=CARTESIAN_POINT('Ctrl Pts',(177.8,0.856168534250961,-104.631980686636));
#19068=CARTESIAN_POINT('Ctrl Pts',(177.8,0.800000000395739,-104.521316838008));
#19069=CARTESIAN_POINT('Ctrl Pts',(177.866666666667,0.915555555555559,-104.876807555876));
#19070=CARTESIAN_POINT('Ctrl Pts',(177.866666666667,0.856146146238362,-104.773601644526));
#19071=CARTESIAN_POINT('Ctrl Pts',(177.868914723125,0.799233317184013,-104.667096072329));
#19072=CARTESIAN_POINT('Ctrl Pts',(177.872973082299,0.743827073473395,-104.557333470599));
#19073=CARTESIAN_POINT('Ctrl Pts',(177.933333333333,0.85777777777778,-104.910066732648));
#19074=CARTESIAN_POINT('Ctrl Pts',(177.933333333333,0.798966141154949,-104.80789927087));
#19075=CARTESIAN_POINT('Ctrl Pts',(177.937829446251,0.742298100117065,-104.702211458022));
#19076=CARTESIAN_POINT('Ctrl Pts',(177.945946164598,0.687654146551051,-104.593350103189));
#19077=CARTESIAN_POINT('Ctrl Pts',(178.,0.800000000000001,-104.943325909419));
#19078=CARTESIAN_POINT('Ctrl Pts',(178.,0.741786136071537,-104.842196897214));
#19079=CARTESIAN_POINT('Ctrl Pts',(178.006744169376,0.685362883050116,-104.737326843716));
#19080=CARTESIAN_POINT('Ctrl Pts',(178.018919246896,0.631481219628706,-104.629366735779));
#19081=CARTESIAN_POINT('Ctrl Pts',(177.8,0.800000000395739,-104.521316838008));
#19082=CARTESIAN_POINT('Ctrl Pts',(177.8,0.856168534250961,-104.631980686636));
#19083=CARTESIAN_POINT('Ctrl Pts',(177.8,0.913326151321774,-104.739304018183));
#19084=CARTESIAN_POINT('Ctrl Pts',(177.8,0.973333333333337,-104.843548379105));
#19085=CARTESIAN_POINT('Ctrl Pts',(178.,0.800000000000001,-104.943325909419));
#19086=CARTESIAN_POINT('Ctrl Pts',(178.,0.741786136071537,-104.842196897214));
#19087=CARTESIAN_POINT('Ctrl Pts',(178.006744169376,0.685362883050116,-104.737326843716));
#19088=CARTESIAN_POINT('Ctrl Pts',(178.018919246896,0.631481219628706,-104.629366735779));
#19089=CARTESIAN_POINT('Origin',(178.6,0.800000000000001,3.35000000000001));
#19090=CARTESIAN_POINT('',(178.6,5.55111512312578E-16,37.8669048105155));
#19091=CARTESIAN_POINT('',(178.6,0.,3.35000000000001));
#19092=CARTESIAN_POINT('',(178.412949235465,0.0221748194567917,38.3827594988839));
#19093=CARTESIAN_POINT('Ctrl Pts',(178.412949235466,0.0221748194567948,
38.3827594988839));
#19094=CARTESIAN_POINT('Ctrl Pts',(178.413479204254,0.0220473729950726,
38.3812667426025));
#19095=CARTESIAN_POINT('Ctrl Pts',(178.414010756786,0.0219200771046594,
38.3797698454647));
#19096=CARTESIAN_POINT('Ctrl Pts',(178.414598464366,0.0217800628456899,
38.3781147939891));
#19097=CARTESIAN_POINT('Ctrl Pts',(178.415213506154,0.0216335365404913,
38.3763827662698));
#19098=CARTESIAN_POINT('Ctrl Pts',(178.415890039171,0.021473078883751,38.3744775538397));
#19099=CARTESIAN_POINT('Ctrl Pts',(178.416671530857,0.0212890957475055,
38.372276994541));
#19100=CARTESIAN_POINT('Ctrl Pts',(178.417481885728,0.0210983174791605,
38.3699951609939));
#19101=CARTESIAN_POINT('Ctrl Pts',(178.418405028268,0.0208822545602319,
38.3673959500167));
#19102=CARTESIAN_POINT('Ctrl Pts',(178.419469999136,0.020635567408783,38.364398541496));
#19103=CARTESIAN_POINT('Ctrl Pts',(178.420583050087,0.0203777431090619,
38.3612658094169));
#19104=CARTESIAN_POINT('Ctrl Pts',(178.421850944588,0.0200864904140129,
38.3576983464094));
#19105=CARTESIAN_POINT('Ctrl Pts',(178.423287112231,0.0197612190513805,
38.3536601223018));
#19106=CARTESIAN_POINT('Ctrl Pts',(178.424806600538,0.0194170767537217,
38.349387616688));
#19107=CARTESIAN_POINT('Ctrl Pts',(178.426514353473,0.0190349038180035,
38.3445884468523));
#19108=CARTESIAN_POINT('Ctrl Pts',(178.428406028054,0.0186194852750736,
38.3392774857728));
#19109=CARTESIAN_POINT('Ctrl Pts',(178.430450936267,0.0181704160751999,
38.3335363144092));
#19110=CARTESIAN_POINT('Ctrl Pts',(178.432710630262,0.0176825938577037,
38.3271975204197));
#19111=CARTESIAN_POINT('Ctrl Pts',(178.435158387722,0.0171671679971481,
38.32033971997));
#19112=CARTESIAN_POINT('Ctrl Pts',(178.437934875626,0.016582521155743,38.3125609263962));
#19113=CARTESIAN_POINT('Ctrl Pts',(178.440953083125,0.015962561625803,38.3041151608828));
#19114=CARTESIAN_POINT('Ctrl Pts',(178.444150464042,0.0153275064450717,
38.2951822723775));
#19115=CARTESIAN_POINT('Ctrl Pts',(178.44910337839,0.0143437719454808,38.2813447494813));
#19116=CARTESIAN_POINT('Ctrl Pts',(178.454484765716,0.0133254516247874,
38.2663432690601));
#19117=CARTESIAN_POINT('Ctrl Pts',(178.460013155354,0.0123429151425505,
38.2509734080791));
#19118=CARTESIAN_POINT('Ctrl Pts',(178.463544800827,0.0117152512572958,
38.2411548345874));
#19119=CARTESIAN_POINT('Ctrl Pts',(178.467135313259,0.0111019336470022,
38.2311887559332));
#19120=CARTESIAN_POINT('Ctrl Pts',(178.47071857634,0.0105151594258905,38.2212593969797));
#19121=CARTESIAN_POINT('Ctrl Pts',(178.474077885478,0.00996505859359832,
38.2119506229607));
#19122=CARTESIAN_POINT('Ctrl Pts',(178.477430307718,0.00943826380387005,
38.2026754958373));
#19123=CARTESIAN_POINT('Ctrl Pts',(178.480737807519,0.00893961706793955,
38.1935386635314));
#19124=CARTESIAN_POINT('Ctrl Pts',(178.483628038754,0.00850387875849878,
38.1855545184929));
#19125=CARTESIAN_POINT('Ctrl Pts',(178.486483947384,0.00808954576042137,
38.1776759878461));
#19126=CARTESIAN_POINT('Ctrl Pts',(178.489295950413,0.00769664054413144,
38.1699285342222));
#19127=CARTESIAN_POINT('Ctrl Pts',(178.491938939309,0.00732735071308687,
38.1626467376943));
#19128=CARTESIAN_POINT('Ctrl Pts',(178.494543049409,0.00697694605925282,
38.1554809706184));
#19129=CARTESIAN_POINT('Ctrl Pts',(178.497116210763,0.00664325432236268,
38.1484081971558));
#19130=CARTESIAN_POINT('Ctrl Pts',(178.499585585533,0.00632302179792544,
38.1416206988443));
#19131=CARTESIAN_POINT('Ctrl Pts',(178.502026366902,0.00601814542141101,
38.1349190820401));
#19132=CARTESIAN_POINT('Ctrl Pts',(178.504462009072,0.00572517836110786,
38.1282375070276));
#19133=CARTESIAN_POINT('Ctrl Pts',(178.506947353139,0.00542623299299849,
38.1214195872942));
#19134=CARTESIAN_POINT('Ctrl Pts',(178.509430134168,0.00513933094283238,
38.1146148150562));
#19135=CARTESIAN_POINT('Ctrl Pts',(178.511941401537,0.00486121762499003,
38.107736476015));
#19136=CARTESIAN_POINT('Ctrl Pts',(178.514532859657,0.00457422348627795,
38.10063849522));
#19137=CARTESIAN_POINT('Ctrl Pts',(178.517154590214,0.00429665299515969,
38.0934623655918));
#19138=CARTESIAN_POINT('Ctrl Pts',(178.519820345447,0.00402812675590003,
38.0861692115369));
#19139=CARTESIAN_POINT('Ctrl Pts',(178.522634239058,0.0037446782757912,
38.0784707704542));
#19140=CARTESIAN_POINT('Ctrl Pts',(178.525497078762,0.0034713852594164,
38.0706422517076));
#19141=CARTESIAN_POINT('Ctrl Pts',(178.528404163057,0.00321016815445696,
38.0626954690102));
#19142=CARTESIAN_POINT('Ctrl Pts',(178.531533001884,0.00292902521621764,
38.0541424998719));
#19143=CARTESIAN_POINT('Ctrl Pts',(178.534712934459,0.00266197609671292,
38.0454529879565));
#19144=CARTESIAN_POINT('Ctrl Pts',(178.537916542669,0.00241261022643413,
38.0367007916547));
#19145=CARTESIAN_POINT('Ctrl Pts',(178.541525054487,0.00213172703747435,
38.0268424064438));
#19146=CARTESIAN_POINT('Ctrl Pts',(178.54516332883,0.0018734476443256,38.0169052582021));
#19147=CARTESIAN_POINT('Ctrl Pts',(178.548768955785,0.00164207268377403,
38.0070583420493));
#19148=CARTESIAN_POINT('Ctrl Pts',(178.555559822268,0.00120629924286804,
37.9885125818511));
#19149=CARTESIAN_POINT('Ctrl Pts',(178.562232482599,0.000869036079380652,
37.9702933136435));
#19150=CARTESIAN_POINT('Ctrl Pts',(178.568284359434,0.000628923375684654,
37.9537634911092));
#19151=CARTESIAN_POINT('Ctrl Pts',(178.571379493236,0.000506121645651807,
37.9453095827024));
#19152=CARTESIAN_POINT('Ctrl Pts',(178.574311652108,0.00040793334416573,
37.9372992319626));
#19153=CARTESIAN_POINT('Ctrl Pts',(178.577024252739,0.000329996162289015,
37.9298861298665));
#19154=CARTESIAN_POINT('Ctrl Pts',(178.579468756696,0.000259761809582353,
37.9232056929462));
#19155=CARTESIAN_POINT('Ctrl Pts',(178.581734725427,0.000205884912835238,
37.9170109178203));
#19156=CARTESIAN_POINT('Ctrl Pts',(178.583795075103,0.000164141583355315,
37.9113755217763));
#19157=CARTESIAN_POINT('Ctrl Pts',(178.585722017181,0.000125101133586624,
37.9061050175084));
#19158=CARTESIAN_POINT('Ctrl Pts',(178.587468956389,9.66253259402746E-5,
37.9013242110118));
#19159=CARTESIAN_POINT('Ctrl Pts',(178.589029536688,7.5222952356846E-5,
37.897050537843));
#19160=CARTESIAN_POINT('Ctrl Pts',(178.590481114415,5.53154802371808E-5,
37.893075369896));
#19161=CARTESIAN_POINT('Ctrl Pts',(178.591771417204,4.15083062714315E-5,
37.8895390806041));
#19162=CARTESIAN_POINT('Ctrl Pts',(178.592910673892,3.1412207123438E-5,
37.886413974605));
#19163=CARTESIAN_POINT('Ctrl Pts',(178.59401538403,2.16222596854959E-5,
37.8833836335772));
#19164=CARTESIAN_POINT('Ctrl Pts',(178.59497796706,1.53159280371486E-5,
37.8807402004026));
#19165=CARTESIAN_POINT('Ctrl Pts',(178.595823866029,1.09001335970582E-5,
37.8784145222615));
#19166=CARTESIAN_POINT('Ctrl Pts',(178.596647541578,6.6003507133465E-6,
37.8761499442337));
#19167=CARTESIAN_POINT('Ctrl Pts',(178.597360497011,4.09626587143205E-6,
37.8741868830685));
#19168=CARTESIAN_POINT('Ctrl Pts',(178.598003120417,2.49220892567514E-6,
37.8724154152598));
#19169=CARTESIAN_POINT('Ctrl Pts',(178.598625651521,9.38304521417067E-7,
37.8706993342708));
#19170=CARTESIAN_POINT('Ctrl Pts',(178.59918213145,2.32998665909085E-7,
37.8691631867779));
#19171=CARTESIAN_POINT('Ctrl Pts',(178.599726292382,4.68224145011575E-8,
37.867660612874));
#19172=CARTESIAN_POINT('Ctrl Pts',(178.599817733235,1.55373403223607E-8,
37.8674081202189));
#19173=CARTESIAN_POINT('Ctrl Pts',(178.599908867247,6.6612116756507E-16,
37.867156463647));
#19174=CARTESIAN_POINT('Ctrl Pts',(178.6,6.66133814775094E-16,37.8669048105155));
#19175=CARTESIAN_POINT('',(177.8,0.800000000220449,41.0213168380973));
#19176=CARTESIAN_POINT('Ctrl Pts',(177.8,0.800000000395797,41.0213168380085));
#19177=CARTESIAN_POINT('Ctrl Pts',(177.799999999912,0.62257825368506,40.6717586072261));
#19178=CARTESIAN_POINT('Ctrl Pts',(177.858376073723,0.4624110846645,40.2928391623376));
#19179=CARTESIAN_POINT('Ctrl Pts',(178.066773051231,0.169426085453293,39.3947605243754));
#19180=CARTESIAN_POINT('Ctrl Pts',(178.240471017511,0.0636522405289915,
38.8685766805066));
#19181=CARTESIAN_POINT('Ctrl Pts',(178.412949235465,0.0221748194567911,
38.3827594988839));
#19182=CARTESIAN_POINT('',(177.8,0.800000000000001,3.35000000000001));
#19183=CARTESIAN_POINT('Origin',(177.8,0.,38.45));
#19184=CARTESIAN_POINT('',(181.549583741031,0.,-101.95));
#19185=CARTESIAN_POINT('',(177.8,0.,-101.95));
#19186=CARTESIAN_POINT('',(181.7625,5.55111512312578E-16,-101.366904810515));
#19187=CARTESIAN_POINT('',(181.656041870516,2.77555756156289E-16,-101.658452405258));
#19188=CARTESIAN_POINT('',(181.7625,5.55111512312578E-16,37.8669048105155));
#19189=CARTESIAN_POINT('',(181.7625,0.,3.35000000000001));
#19190=CARTESIAN_POINT('',(181.549583741031,2.22044604925031E-15,38.45));
#19191=CARTESIAN_POINT('',(181.656041870515,1.38777878078145E-15,38.1584524052577));
#19192=CARTESIAN_POINT('',(178.812916258969,2.22044604925031E-15,38.45));
#19193=CARTESIAN_POINT('',(177.8,2.22044604925031E-15,38.45));
#19194=CARTESIAN_POINT('',(178.706458129484,1.38777878078145E-15,38.1584524052578));
#19195=CARTESIAN_POINT('Origin',(177.8,6.00000000000001,-101.95));
#19196=CARTESIAN_POINT('',(181.549583741031,6.,-107.95));
#19197=CARTESIAN_POINT('',(177.8,6.,-107.95));
#19198=CARTESIAN_POINT('',(181.574975446846,5.93046313286183,-107.949597038478));
#19199=CARTESIAN_POINT('Ctrl Pts',(181.574975446847,5.93046313286183,-107.949597038478));
#19200=CARTESIAN_POINT('Ctrl Pts',(181.574851587102,5.93080231399545,-107.949600969674));
#19201=CARTESIAN_POINT('Ctrl Pts',(181.574726118725,5.93114590045353,-107.949604929021));
#19202=CARTESIAN_POINT('Ctrl Pts',(181.574566383937,5.93158332281071,-107.949609917176));
#19203=CARTESIAN_POINT('Ctrl Pts',(181.574399215445,5.93204110183877,-107.949615137469));
#19204=CARTESIAN_POINT('Ctrl Pts',(181.574194656871,5.93260127070279,-107.949621481053));
#19205=CARTESIAN_POINT('Ctrl Pts',(181.573935264898,5.93331159796672,-107.949629376639));
#19206=CARTESIAN_POINT('Ctrl Pts',(181.573641850187,5.93411509418438,-107.949638307838));
#19207=CARTESIAN_POINT('Ctrl Pts',(181.573278283541,5.93511069786036,-107.949649222747));
#19208=CARTESIAN_POINT('Ctrl Pts',(181.572843534142,5.93630123568595,-107.949661862757));
#19209=CARTESIAN_POINT('Ctrl Pts',(181.5723678608,5.93760384152415,-107.9496756926));
#19210=CARTESIAN_POINT('Ctrl Pts',(181.571807418754,5.9391385869165,-107.94969155866));
#19211=CARTESIAN_POINT('Ctrl Pts',(181.571184449722,5.94084456975789,-107.949708379169));
#19212=CARTESIAN_POINT('Ctrl Pts',(181.570252774797,5.94339593483727,-107.949733534908));
#19213=CARTESIAN_POINT('Ctrl Pts',(181.569182929476,5.94632569724474,-107.949760665181));
#19214=CARTESIAN_POINT('Ctrl Pts',(181.568089299526,5.94932062429873,-107.949785962922));
#19215=CARTESIAN_POINT('Ctrl Pts',(181.567351775576,5.95134034809351,-107.949803023254));
#19216=CARTESIAN_POINT('Ctrl Pts',(181.566604545459,5.95338666560009,-107.949819263662));
#19217=CARTESIAN_POINT('Ctrl Pts',(181.565874294746,5.95538649749657,-107.94983413399));
#19218=CARTESIAN_POINT('Ctrl Pts',(181.565237964273,5.95712912362859,-107.949847091791));
#19219=CARTESIAN_POINT('Ctrl Pts',(181.564614768374,5.95883579007666,-107.949859020331));
#19220=CARTESIAN_POINT('Ctrl Pts',(181.564008582509,5.96049588210055,-107.949869950646));
#19221=CARTESIAN_POINT('Ctrl Pts',(181.563441613107,5.96204857647315,-107.949880173838));
#19222=CARTESIAN_POINT('Ctrl Pts',(181.562889712943,5.96356001028182,-107.949889531659));
#19223=CARTESIAN_POINT('Ctrl Pts',(181.56234018139,5.9650649629533,-107.949898294404));
#19224=CARTESIAN_POINT('Ctrl Pts',(181.5617897477,5.96657238622942,-107.949907071534));
#19225=CARTESIAN_POINT('Ctrl Pts',(181.561238593153,5.9680817889974,-107.949915301922));
#19226=CARTESIAN_POINT('Ctrl Pts',(181.560672630617,5.96963174796805,-107.949923146947));
#19227=CARTESIAN_POINT('Ctrl Pts',(181.56005990152,5.97130978299697,-107.949931640221));
#19228=CARTESIAN_POINT('Ctrl Pts',(181.55942999806,5.97303485537968,-107.949939665741));
#19229=CARTESIAN_POINT('Ctrl Pts',(181.55878590025,5.97479880212237,-107.949947074735));
#19230=CARTESIAN_POINT('Ctrl Pts',(181.558033049521,5.97686058306593,-107.949955734703));
#19231=CARTESIAN_POINT('Ctrl Pts',(181.557261103323,5.97897466126266,-107.949963524226));
#19232=CARTESIAN_POINT('Ctrl Pts',(181.55649893061,5.98106197314285,-107.94997011252));
#19233=CARTESIAN_POINT('Ctrl Pts',(181.555584005774,5.98356761713471,-107.949978021219));
#19234=CARTESIAN_POINT('Ctrl Pts',(181.554684783888,5.98603025599236,-107.949984153345));
#19235=CARTESIAN_POINT('Ctrl Pts',(181.553868772039,5.98826500948326,-107.949988524155));
#19236=CARTESIAN_POINT('Ctrl Pts',(181.553239803013,5.98998752212496,-107.949991893107));
#19237=CARTESIAN_POINT('Ctrl Pts',(181.552661056841,5.99157249064165,-107.949994240505));
#19238=CARTESIAN_POINT('Ctrl Pts',(181.552156544722,5.99295415655168,-107.949995863006));
#19239=CARTESIAN_POINT('Ctrl Pts',(181.551698261038,5.99420922044089,-107.949997336838));
#19240=CARTESIAN_POINT('Ctrl Pts',(181.551301549687,5.99529565802532,-107.949998223794));
#19241=CARTESIAN_POINT('Ctrl Pts',(181.550971624754,5.99619919007983,-107.949998796154));
#19242=CARTESIAN_POINT('Ctrl Pts',(181.550662042814,5.99704701083767,-107.949999333221));
#19243=CARTESIAN_POINT('Ctrl Pts',(181.550411466451,5.9977332351975,-107.94999959747));
#19244=CARTESIAN_POINT('Ctrl Pts',(181.550208860189,5.99828808589276,-107.949999755779));
#19245=CARTESIAN_POINT('Ctrl Pts',(181.550019269662,5.99880729213513,-107.949999903919));
#19246=CARTESIAN_POINT('Ctrl Pts',(181.549871769533,5.9992112272231,-107.949999958751));
#19247=CARTESIAN_POINT('Ctrl Pts',(181.549741547127,5.99956784464628,-107.949999984437));
#19248=CARTESIAN_POINT('Ctrl Pts',(181.549687047567,5.99971709310156,-107.949999995187));
#19249=CARTESIAN_POINT('Ctrl Pts',(181.549635368945,5.99985861598446,-107.95));
#19250=CARTESIAN_POINT('Ctrl Pts',(181.549583741031,6.,-107.95));
#19251=CARTESIAN_POINT('',(182.343580753104,3.32063326422071,-107.318518780371));
#19252=CARTESIAN_POINT('Ctrl Pts',(182.343580753104,3.32063326422059,-107.318518780371));
#19253=CARTESIAN_POINT('Ctrl Pts',(182.305122859126,3.66165108343612,-107.488716899907));
#19254=CARTESIAN_POINT('Ctrl Pts',(182.21306296514,4.03399937391406,-107.632528959141));
#19255=CARTESIAN_POINT('Ctrl Pts',(181.945261097542,4.92124458677734,-107.875508608848));
#19256=CARTESIAN_POINT('Ctrl Pts',(181.752371143193,5.4446775876699,-107.943966659521));
#19257=CARTESIAN_POINT('Ctrl Pts',(181.574975446846,5.93046313286183,-107.949597038478));
#19258=CARTESIAN_POINT('',(182.3625,3.00667409058086,-107.15));
#19259=CARTESIAN_POINT('Ctrl Pts',(182.3625,3.00667409058087,-107.15));
#19260=CARTESIAN_POINT('Ctrl Pts',(182.3625,3.10780310278612,-107.208213863928));
#19261=CARTESIAN_POINT('Ctrl Pts',(182.355755830624,3.21267315628447,-107.26463711695));
#19262=CARTESIAN_POINT('Ctrl Pts',(182.343580753104,3.32063326422071,-107.318518780371));
#19263=CARTESIAN_POINT('',(182.3625,0.800000000000001,-104.943325909419));
#19264=CARTESIAN_POINT('Origin',(182.3625,6.00000000000001,-101.95));
#19265=CARTESIAN_POINT('',(182.343580753256,0.631481220303021,-104.62936673713));
#19266=CARTESIAN_POINT('Ctrl Pts',(182.343580753256,0.631481220303025,-104.62936673713));
#19267=CARTESIAN_POINT('Ctrl Pts',(182.355987338329,0.686387436939596,-104.739379693196));
#19268=CARTESIAN_POINT('Ctrl Pts',(182.3625,0.743322320630639,-104.844865554069));
#19269=CARTESIAN_POINT('Ctrl Pts',(182.3625,0.799999999999998,-104.943325909419));
#19270=CARTESIAN_POINT('',(181.5749753816,0.000402959451920593,-102.019536688494));
#19271=CARTESIAN_POINT('Ctrl Pts',(181.5749753816,0.000402959451920593,
-102.019536688494));
#19272=CARTESIAN_POINT('Ctrl Pts',(181.765769469498,0.0064585754895931,
-102.542012763284));
#19273=CARTESIAN_POINT('Ctrl Pts',(181.990548412461,0.0977146252752476,
-103.158388759139));
#19274=CARTESIAN_POINT('Ctrl Pts',(182.224838707103,0.341969925937946,-103.971322135667));
#19275=CARTESIAN_POINT('Ctrl Pts',(182.308539856551,0.47640526231532,-104.318648468817));
#19276=CARTESIAN_POINT('Ctrl Pts',(182.343580753256,0.631481220303202,-104.629366737131));
#19277=CARTESIAN_POINT('Ctrl Pts',(181.549583741031,0.,-101.95));
#19278=CARTESIAN_POINT('Ctrl Pts',(181.54970760812,0.,-101.950339212386));
#19279=CARTESIAN_POINT('Ctrl Pts',(181.549833083808,2.29071906254038E-8,
-101.950682830141));
#19280=CARTESIAN_POINT('Ctrl Pts',(181.549992825092,1.04587385862942E-7,
-101.951120289523));
#19281=CARTESIAN_POINT('Ctrl Pts',(181.550160000382,1.90068796205335E-7,
-101.951578107295));
#19282=CARTESIAN_POINT('Ctrl Pts',(181.550364564865,3.38981443109131E-7,
-101.952138321158));
#19283=CARTESIAN_POINT('Ctrl Pts',(181.550623961395,6.76258333776047E-7,
-101.952848701379));
#19284=CARTESIAN_POINT('Ctrl Pts',(181.550917381295,1.05777365854045E-6,
-101.953652257592));
#19285=CARTESIAN_POINT('Ctrl Pts',(181.551280951416,1.68214207260373E-6,
-101.954647931466));
#19286=CARTESIAN_POINT('Ctrl Pts',(181.551715702461,2.84071918610351E-6,
-101.955838546237));
#19287=CARTESIAN_POINT('Ctrl Pts',(181.552191377746,4.10835615815435E-6,
-101.957141236654));
#19288=CARTESIAN_POINT('Ctrl Pts',(181.552751819603,6.03030069600252E-6,
-101.958676074583));
#19289=CARTESIAN_POINT('Ctrl Pts',(181.553374786724,8.98242465474652E-6,
-101.960382148871));
#19290=CARTESIAN_POINT('Ctrl Pts',(181.554306457762,1.33974383844118E-5,
-101.962933647896));
#19291=CARTESIAN_POINT('Ctrl Pts',(181.555376295022,2.02235012763771E-5,
-101.965863539379));
#19292=CARTESIAN_POINT('Ctrl Pts',(181.556469915917,2.9637200332111E-5,
-101.968858566372));
#19293=CARTESIAN_POINT('Ctrl Pts',(181.557207433796,3.59856263709023E-5,
-101.970878357661));
#19294=CARTESIAN_POINT('Ctrl Pts',(181.557954657433,4.34621306637084E-5,
-101.97292472978));
#19295=CARTESIAN_POINT('Ctrl Pts',(181.558684902273,5.17698706108405E-5,
-101.974924601646));
#19296=CARTESIAN_POINT('Ctrl Pts',(181.559321227784,5.90091232076345E-5,
-101.97666726303));
#19297=CARTESIAN_POINT('Ctrl Pts',(181.559944419184,6.68608083979287E-5,
-101.978373953766));
#19298=CARTESIAN_POINT('Ctrl Pts',(181.560550601505,7.51708677384499E-5,
-101.980034060035));
#19299=CARTESIAN_POINT('Ctrl Pts',(181.561117567921,8.29433223074671E-5,
-101.98158676863));
#19300=CARTESIAN_POINT('Ctrl Pts',(181.561669465921,9.11028932043242E-5,
-101.983098207949));
#19301=CARTESIAN_POINT('Ctrl Pts',(181.562218996326,9.9782376472568E-5,
-101.984603158254));
#19302=CARTESIAN_POINT('Ctrl Pts',(181.562769428947,0.000108476109649939,
-101.986110579374));
#19303=CARTESIAN_POINT('Ctrl Pts',(181.56332058345,0.000117739478919532,
-101.987619972111));
#19304=CARTESIAN_POINT('Ctrl Pts',(181.563886546778,0.000127858198572639,
-101.989169912371));
#19305=CARTESIAN_POINT('Ctrl Pts',(181.564499277062,0.000138813053173701,
-101.990847928046));
#19306=CARTESIAN_POINT('Ctrl Pts',(181.565129182704,0.000150780753699223,
-101.992572970802));
#19307=CARTESIAN_POINT('Ctrl Pts',(181.56577328316,0.000163815454714999,
-101.994336876537));
#19308=CARTESIAN_POINT('Ctrl Pts',(181.566526137782,0.000179051020544146,
-101.99639861174));
#19309=CARTESIAN_POINT('Ctrl Pts',(181.567298088538,0.0001957630484375,
-101.998512628489));
#19310=CARTESIAN_POINT('Ctrl Pts',(181.568060265242,0.000213365986056147,
-102.0005998647));
#19311=CARTESIAN_POINT('Ctrl Pts',(181.568975191389,0.000234496765571556,
-102.003105408326));
#19312=CARTESIAN_POINT('Ctrl Pts',(181.569874413831,0.000256905535015469,
-102.005567926382));
#19313=CARTESIAN_POINT('Ctrl Pts',(181.57069042421,0.000278434394754612,
-102.007802553675));
#19314=CARTESIAN_POINT('Ctrl Pts',(181.571319393029,0.000295028523743357,
-102.009524971582));
#19315=CARTESIAN_POINT('Ctrl Pts',(181.571898137643,0.000311050051264457,
-102.011109842215));
#19316=CARTESIAN_POINT('Ctrl Pts',(181.572402646459,0.000325440246225384,
-102.012491415757));
#19317=CARTESIAN_POINT('Ctrl Pts',(181.572860927247,0.000338511870882684,
-102.013746396029));
#19318=CARTESIAN_POINT('Ctrl Pts',(181.57325763423,0.000350216032188715,
-102.014832754664));
#19319=CARTESIAN_POINT('Ctrl Pts',(181.573587553363,0.000360114993102734,
-102.015736217068));
#19320=CARTESIAN_POINT('Ctrl Pts',(181.573897129891,0.000369403590350718,
-102.016583972552));
#19321=CARTESIAN_POINT('Ctrl Pts',(181.574147699568,0.000377092172797711,
-102.017270139883));
#19322=CARTESIAN_POINT('Ctrl Pts',(181.574350298267,0.000383364144085796,
-102.017824942027));
#19323=CARTESIAN_POINT('Ctrl Pts',(181.574539881751,0.000389233195429729,
-102.018344102929));
#19324=CARTESIAN_POINT('Ctrl Pts',(181.574687374055,0.000393859622541619,
-102.01874800007));
#19325=CARTESIAN_POINT('Ctrl Pts',(181.574817588547,0.000397966817764051,
-102.019104583318));
#19326=CARTESIAN_POINT('Ctrl Pts',(181.574872083688,0.000399685690829952,
-102.019253814438));
#19327=CARTESIAN_POINT('Ctrl Pts',(181.574923757996,0.000401320969685316,
-102.019395320917));
#19328=CARTESIAN_POINT('Ctrl Pts',(181.5749753816,0.000402959451920815,
-102.019536688494));
#19329=CARTESIAN_POINT('Ctrl Pts',(178.412949792571,6.06724207026202,44.4278253145154));
#19330=CARTESIAN_POINT('Ctrl Pts',(178.42318867301,6.09608178690105,44.4302875443684));
#19331=CARTESIAN_POINT('Ctrl Pts',(178.514957272365,6.35253399018344,44.4503778941236));
#19332=CARTESIAN_POINT('Ctrl Pts',(178.592152189615,6.56142469489367,44.45));
#19333=CARTESIAN_POINT('Ctrl Pts',(178.6,6.58309518948451,44.45));
#19334=CARTESIAN_POINT('Ctrl Pts',(178.537808064946,6.02164914272028,44.4350825564341));
#19335=CARTESIAN_POINT('Ctrl Pts',(178.545154992406,6.04220443093549,44.4361237601754));
#19336=CARTESIAN_POINT('Ctrl Pts',(178.609869985354,6.22405274576398,44.452422433776));
#19337=CARTESIAN_POINT('Ctrl Pts',(178.665385913285,6.37331287412804,44.45));
#19338=CARTESIAN_POINT('Ctrl Pts',(178.670972086323,6.38873012632301,44.45));
#19339=CARTESIAN_POINT('Ctrl Pts',(178.662666337321,5.97605621517853,44.4423397983527));
#19340=CARTESIAN_POINT('Ctrl Pts',(178.667058000585,5.98825131680075,44.4425732795651));
#19341=CARTESIAN_POINT('Ctrl Pts',(178.706720690063,6.09746305536317,44.4476687386033));
#19342=CARTESIAN_POINT('Ctrl Pts',(178.738619636954,6.18520105336241,44.45));
#19343=CARTESIAN_POINT('Ctrl Pts',(178.741944172646,6.1943650631615,44.45));
#19344=CARTESIAN_POINT('Ctrl Pts',(178.787524609695,5.93046328763679,44.4495970402714));
#19345=CARTESIAN_POINT('Ctrl Pts',(178.788941720953,5.93434394615833,44.449642017998));
#19346=CARTESIAN_POINT('Ctrl Pts',(178.8015714622,5.96893024314017,44.4500079385574));
#19347=CARTESIAN_POINT('Ctrl Pts',(178.811853360624,5.99708923259677,44.45));
#19348=CARTESIAN_POINT('Ctrl Pts',(178.812916258969,6.,44.45));
#19349=CARTESIAN_POINT('',(178.6,6.58309518948451,44.45));
#19350=CARTESIAN_POINT('',(178.412949792571,6.06724207026202,44.4278253145154));
#19351=CARTESIAN_POINT('Ctrl Pts',(178.6,6.58309518948452,44.45));
#19352=CARTESIAN_POINT('Ctrl Pts',(178.599458517973,6.58159997199468,44.45));
#19353=CARTESIAN_POINT('Ctrl Pts',(178.598915520309,6.58010061762004,44.4499994906954));
#19354=CARTESIAN_POINT('Ctrl Pts',(178.598314514906,6.57844323223622,44.4499982244605));
#19355=CARTESIAN_POINT('Ctrl Pts',(178.597685564613,6.57670878356453,44.4499968993497));
#19356=CARTESIAN_POINT('Ctrl Pts',(178.596993094733,6.57480128952343,44.449994749902));
#19357=CARTESIAN_POINT('Ctrl Pts',(178.596192260443,6.57259867771452,44.4499909381484));
#19358=CARTESIAN_POINT('Ctrl Pts',(178.595361861441,6.57031475122541,44.4499869856747));
#19359=CARTESIAN_POINT('Ctrl Pts',(178.594415017345,6.56771370326992,44.4499812514669));
#19360=CARTESIAN_POINT('Ctrl Pts',(178.593322018501,6.56471476414272,44.4499721273664));
#19361=CARTESIAN_POINT('Ctrl Pts',(178.59217970018,6.561580503641,44.4499625915584));
#19362=CARTESIAN_POINT('Ctrl Pts',(178.590877823263,6.55801186637361,44.4499493490856));
#19363=CARTESIAN_POINT('Ctrl Pts',(178.589403093044,6.55397282717115,44.449929812898));
#19364=CARTESIAN_POINT('Ctrl Pts',(178.587842862039,6.54969961562671,44.4499091440561));
#19365=CARTESIAN_POINT('Ctrl Pts',(178.586089262768,6.54490018007633,44.4498814053308));
#19366=CARTESIAN_POINT('Ctrl Pts',(178.584147685166,6.53958934065723,44.4498429246511));
#19367=CARTESIAN_POINT('Ctrl Pts',(178.582048978208,6.53384870189507,44.4498013297799));
#19368=CARTESIAN_POINT('Ctrl Pts',(178.579730794754,6.52751097601296,44.4497471216981));
#19369=CARTESIAN_POINT('Ctrl Pts',(178.57722196257,6.52065463592149,44.449675659884));
#19370=CARTESIAN_POINT('Ctrl Pts',(178.574377026696,6.51287976440619,44.4495946244604));
#19371=CARTESIAN_POINT('Ctrl Pts',(178.571287228746,6.50443881327361,44.4494912617698));
#19372=CARTESIAN_POINT('Ctrl Pts',(178.56801862387,6.49551119955545,44.4493604891292));
#19373=CARTESIAN_POINT('Ctrl Pts',(178.56294420415,6.48165132329992,44.4491574681794));
#19374=CARTESIAN_POINT('Ctrl Pts',(178.557440622755,6.46662341589086,44.4488871027284));
#19375=CARTESIAN_POINT('Ctrl Pts',(178.551802564766,6.45122671631941,44.4485468096717));
#19376=CARTESIAN_POINT('Ctrl Pts',(178.548206420165,6.44140617915121,44.448329759219));
#19377=CARTESIAN_POINT('Ctrl Pts',(178.544556616115,6.43143843660386,44.4480847826414));
#19378=CARTESIAN_POINT('Ctrl Pts',(178.540921148225,6.4215076975126,44.4478155734711));
#19379=CARTESIAN_POINT('Ctrl Pts',(178.537512897078,6.41219762961454,44.4475631898739));
#19380=CARTESIAN_POINT('Ctrl Pts',(178.534117745962,6.40292145768546,44.4472896528906));
#19381=CARTESIAN_POINT('Ctrl Pts',(178.530774442786,6.39378380888695,44.4469992611216));
#19382=CARTESIAN_POINT('Ctrl Pts',(178.527853421831,6.38580030807624,44.4467455478335));
#19383=CARTESIAN_POINT('Ctrl Pts',(178.52497197727,6.3779225584153,44.4464790605755));
#19384=CARTESIAN_POINT('Ctrl Pts',(178.522139765614,6.37017599734817,44.4462020999102));
#19385=CARTESIAN_POINT('Ctrl Pts',(178.519478224497,6.36289624805762,44.4459418290378));
#19386=CARTESIAN_POINT('Ctrl Pts',(178.5168602412,6.35573258653662,44.445672374142));
#19387=CARTESIAN_POINT('Ctrl Pts',(178.514277799497,6.34866200275349,44.445394056013));
#19388=CARTESIAN_POINT('Ctrl Pts',(178.511798987803,6.34187515225487,44.4451269064267));
#19389=CARTESIAN_POINT('Ctrl Pts',(178.509353003695,6.33517429878812,44.4448516471374));
#19390=CARTESIAN_POINT('Ctrl Pts',(178.506916323581,6.328493643819,44.4445661893035));
#19391=CARTESIAN_POINT('Ctrl Pts',(178.504429011938,6.32167417219901,44.4442747999703));
#19392=CARTESIAN_POINT('Ctrl Pts',(178.5019486018,6.31486802670454,44.4439724785344));
#19393=CARTESIAN_POINT('Ctrl Pts',(178.499444072893,6.30798842616424,44.4436551552934));
#19394=CARTESIAN_POINT('Ctrl Pts',(178.496859698675,6.30088950140187,44.4433277156695));
#19395=CARTESIAN_POINT('Ctrl Pts',(178.494249717861,6.29371255464342,44.4429842542725));
#19396=CARTESIAN_POINT('Ctrl Pts',(178.491600486335,6.28641868903367,44.4426219435754));
#19397=CARTESIAN_POINT('Ctrl Pts',(178.488804030965,6.27871948666037,44.4422394984456));
#19398=CARTESIAN_POINT('Ctrl Pts',(178.485963962915,6.27089032428992,44.4418360005005));
#19399=CARTESIAN_POINT('Ctrl Pts',(178.483084978334,6.26294302810835,44.4414106883969));
#19400=CARTESIAN_POINT('Ctrl Pts',(178.479986370237,6.25438947194786,44.4409529313334));
#19401=CARTESIAN_POINT('Ctrl Pts',(178.476842858534,6.24569952323156,44.4404698404418));
#19402=CARTESIAN_POINT('Ctrl Pts',(178.473681436809,6.23694709174931,44.4399643160253));
#19403=CARTESIAN_POINT('Ctrl Pts',(178.470120305089,6.22708805866677,44.4393948763265));
#19404=CARTESIAN_POINT('Ctrl Pts',(178.466536752565,6.21715051315623,44.4387968743326));
#19405=CARTESIAN_POINT('Ctrl Pts',(178.46299166798,6.20730357410851,44.4381806372635));
#19406=CARTESIAN_POINT('Ctrl Pts',(178.456316782679,6.18876320161894,44.4370203513363));
#19407=CARTESIAN_POINT('Ctrl Pts',(178.44978125028,6.17055048437432,44.4357930266506));
#19408=CARTESIAN_POINT('Ctrl Pts',(178.443867806725,6.15402796694876,44.4346162999984));
#19409=CARTESIAN_POINT('Ctrl Pts',(178.440842493664,6.14557506005742,44.4340142875707));
#19410=CARTESIAN_POINT('Ctrl Pts',(178.437980411313,6.13756619273647,44.4334264231729));
#19411=CARTESIAN_POINT('Ctrl Pts',(178.435335029566,6.13015512599593,44.4328700067777));
#19412=CARTESIAN_POINT('Ctrl Pts',(178.432951184304,6.12347675666169,44.4323686006615));
#19413=CARTESIAN_POINT('Ctrl Pts',(178.430743513708,6.11728446376527,44.4318928704646));
#19414=CARTESIAN_POINT('Ctrl Pts',(178.428737104348,6.11165195374683,44.4314531467548));
#19415=CARTESIAN_POINT('Ctrl Pts',(178.42686063372,6.10638421535628,44.4310419003549));
#19416=CARTESIAN_POINT('Ctrl Pts',(178.425160333831,6.10160651578871,44.4306622290609));
#19417=CARTESIAN_POINT('Ctrl Pts',(178.423641481701,6.09733622922153,44.4303189559555));
#19418=CARTESIAN_POINT('Ctrl Pts',(178.422228714802,6.09336420364257,44.4299996589872));
#19419=CARTESIAN_POINT('Ctrl Pts',(178.420972968814,6.08983130045456,44.4297118814688));
#19420=CARTESIAN_POINT('Ctrl Pts',(178.419863784619,6.08670972753893,44.4294555432534));
#19421=CARTESIAN_POINT('Ctrl Pts',(178.418788240371,6.0836828273976,44.4292069794038));
#19422=CARTESIAN_POINT('Ctrl Pts',(178.417850600654,6.08104296971711,44.4289880063072));
#19423=CARTESIAN_POINT('Ctrl Pts',(178.417025912301,6.07872086557605,44.4287942496133));
#19424=CARTESIAN_POINT('Ctrl Pts',(178.416222893088,6.07645977599809,44.4286055839832));
#19425=CARTESIAN_POINT('Ctrl Pts',(178.415527051897,6.07450019982907,44.4284408442171));
#19426=CARTESIAN_POINT('Ctrl Pts',(178.414899175626,6.07273203935875,44.4282915166029));
#19427=CARTESIAN_POINT('Ctrl Pts',(178.41429092292,6.07101914074931,44.4281468560549));
#19428=CARTESIAN_POINT('Ctrl Pts',(178.413746500949,6.06948601365089,44.4280166669529));
#19429=CARTESIAN_POINT('Ctrl Pts',(178.413213947771,6.06798608491948,44.4278887906975));
#19430=CARTESIAN_POINT('Ctrl Pts',(178.413125702731,6.06773754397356,44.427867601367));
#19431=CARTESIAN_POINT('Ctrl Pts',(178.413037745286,6.06748980548983,44.4278464652458));
#19432=CARTESIAN_POINT('Ctrl Pts',(178.412949792571,6.06724207026203,44.4278253145154));
#19433=CARTESIAN_POINT('',(178.787524609695,5.93046328763679,44.4495970402714));
#19434=CARTESIAN_POINT('Ctrl Pts',(178.787524609695,5.93046328763679,44.4495970402714));
#19435=CARTESIAN_POINT('Ctrl Pts',(178.662666337321,5.97605621517853,44.4423397983527));
#19436=CARTESIAN_POINT('Ctrl Pts',(178.537808064946,6.02164914272028,44.4350825564341));
#19437=CARTESIAN_POINT('Ctrl Pts',(178.412949792571,6.06724207026202,44.4278253145154));
#19438=CARTESIAN_POINT('',(178.812916258969,6.,44.45));
#19439=CARTESIAN_POINT('Ctrl Pts',(178.787524609695,5.93046328763679,44.4495970402714));
#19440=CARTESIAN_POINT('Ctrl Pts',(178.787648469277,5.93080246830438,44.4496009714535));
#19441=CARTESIAN_POINT('Ctrl Pts',(178.787773937493,5.93114605429704,44.449604930787));
#19442=CARTESIAN_POINT('Ctrl Pts',(178.787933672098,5.93158347612988,44.4496099189249));
#19443=CARTESIAN_POINT('Ctrl Pts',(178.788100840397,5.93204125460652,44.4496151391996));
#19444=CARTESIAN_POINT('Ctrl Pts',(178.788305398756,5.9326014228527,44.4496214827624));
#19445=CARTESIAN_POINT('Ctrl Pts',(178.788564790463,5.9333117493612,44.4496293783222));
#19446=CARTESIAN_POINT('Ctrl Pts',(178.788858204901,5.93411524479927,44.4496383094914));
#19447=CARTESIAN_POINT('Ctrl Pts',(178.789221771224,5.93511084755497,44.4496492243657));
#19448=CARTESIAN_POINT('Ctrl Pts',(178.789656520216,5.93630138422979,44.4496618643344));
#19449=CARTESIAN_POINT('Ctrl Pts',(178.790132193253,5.93760398919225,44.449675694136));
#19450=CARTESIAN_POINT('Ctrl Pts',(178.790692634943,5.93913873356867,44.4496915601474));
#19451=CARTESIAN_POINT('Ctrl Pts',(178.791315603513,5.94084471510306,44.4497083806022));
#19452=CARTESIAN_POINT('Ctrl Pts',(178.792247276602,5.94339607509601,44.4497335362294));
#19453=CARTESIAN_POINT('Ctrl Pts',(178.793317119493,5.94632583079425,44.4497606663719));
#19454=CARTESIAN_POINT('Ctrl Pts',(178.794410746748,5.94932075042631,44.4497859639876));
#19455=CARTESIAN_POINT('Ctrl Pts',(178.795148269123,5.95134046987867,44.4498030242406));
#19456=CARTESIAN_POINT('Ctrl Pts',(178.795895497556,5.95338678275387,44.4498192645702));
#19457=CARTESIAN_POINT('Ctrl Pts',(178.796625746573,5.9553866099923,44.4498341348267));
#19458=CARTESIAN_POINT('Ctrl Pts',(178.797262075683,5.95712923238399,44.449847092567));
#19459=CARTESIAN_POINT('Ctrl Pts',(178.797885270207,5.95883589505943,44.4498590210502));
#19460=CARTESIAN_POINT('Ctrl Pts',(178.798491454741,5.96049598344251,44.4498699513136));
#19461=CARTESIAN_POINT('Ctrl Pts',(178.799058423271,5.96204867543337,44.4498801744635));
#19462=CARTESIAN_POINT('Ctrl Pts',(178.799610322583,5.96356010691652,44.4498895322452));
#19463=CARTESIAN_POINT('Ctrl Pts',(178.800159853383,5.96506505753999,44.4498982949543));
#19464=CARTESIAN_POINT('Ctrl Pts',(178.800710286014,5.96657247792421,44.4499070720438));
#19465=CARTESIAN_POINT('Ctrl Pts',(178.801261439609,5.96808187810208,44.4499153023956));
#19466=CARTESIAN_POINT('Ctrl Pts',(178.801827401211,5.96963183453364,44.449923147385));
#19467=CARTESIAN_POINT('Ctrl Pts',(178.802440129662,5.97130986781118,44.4499316406258));
#19468=CARTESIAN_POINT('Ctrl Pts',(178.803070032518,5.97303493856084,44.4499396661149));
#19469=CARTESIAN_POINT('Ctrl Pts',(178.803714129678,5.97479888354565,44.4499470750774));
#19470=CARTESIAN_POINT('Ctrl Pts',(178.804466980332,5.97686066430854,44.4499557350166));
#19471=CARTESIAN_POINT('Ctrl Pts',(178.805238926428,5.97897474224762,44.4499635245097));
#19472=CARTESIAN_POINT('Ctrl Pts',(178.806001098802,5.98106205322472,44.4499701127732));
#19473=CARTESIAN_POINT('Ctrl Pts',(178.806916020284,5.9835676880624,44.4499780214092));
#19474=CARTESIAN_POINT('Ctrl Pts',(178.807815238561,5.98603031706659,44.449984153484));
#19475=CARTESIAN_POINT('Ctrl Pts',(178.808631246937,5.98826506107557,44.4499885242564));
#19476=CARTESIAN_POINT('Ctrl Pts',(178.809260214051,5.98998756850614,44.4499918931828));
#19477=CARTESIAN_POINT('Ctrl Pts',(178.809838958277,5.99157253171875,44.4499942405612));
#19478=CARTESIAN_POINT('Ctrl Pts',(178.810343468533,5.99295419255149,44.4499958630484));
#19479=CARTESIAN_POINT('Ctrl Pts',(178.810801750615,5.99420925207889,44.4499973368673));
#19480=CARTESIAN_POINT('Ctrl Pts',(178.811198460408,5.99529568542398,44.4499982238154));
#19481=CARTESIAN_POINT('Ctrl Pts',(178.811528383922,5.99619921362319,44.4499987961685));
#19482=CARTESIAN_POINT('Ctrl Pts',(178.811837964558,5.99704703083499,44.4499993332306));
#19483=CARTESIAN_POINT('Ctrl Pts',(178.81208853973,5.99773325196068,44.4499995974758));
#19484=CARTESIAN_POINT('Ctrl Pts',(178.812291145002,5.99828809997737,44.4499997557832));
#19485=CARTESIAN_POINT('Ctrl Pts',(178.812480734631,5.99880730379097,44.4499999039207));
#19486=CARTESIAN_POINT('Ctrl Pts',(178.812628234028,5.99921123690189,44.4499999587523));
#19487=CARTESIAN_POINT('Ctrl Pts',(178.812758455955,5.99956785304632,44.4499999844374));
#19488=CARTESIAN_POINT('Ctrl Pts',(178.812812954392,5.99971709843905,44.4499999951867));
#19489=CARTESIAN_POINT('Ctrl Pts',(178.812864632032,5.99985861864849,44.45));
#19490=CARTESIAN_POINT('Ctrl Pts',(178.812916258969,6.,44.45));
#19491=CARTESIAN_POINT('',(178.706458129484,6.29154759474226,44.45));
#19492=CARTESIAN_POINT('Ctrl Pts',(178.787524038921,0.00040297784403398,
38.5195382753398));
#19493=CARTESIAN_POINT('Ctrl Pts',(178.788055467441,0.000386110442137109,
38.5180829960178));
#19494=CARTESIAN_POINT('Ctrl Pts',(178.789728852842,0.000327539963165485,
38.5135006260165));
#19495=CARTESIAN_POINT('Ctrl Pts',(178.796662726497,0.000156711167295762,
38.494512252932));
#19496=CARTESIAN_POINT('Ctrl Pts',(178.802273531769,5.97527433101154E-5,
38.4791464222591));
#19497=CARTESIAN_POINT('Ctrl Pts',(178.808321057158,7.82364703110596E-6,
38.4625844223785));
#19498=CARTESIAN_POINT('Ctrl Pts',(178.811886047181,-2.86362915729096E-7,
38.4528212764702));
#19499=CARTESIAN_POINT('Ctrl Pts',(178.81256195152,2.22118770383678E-15,
38.4509702776198));
#19500=CARTESIAN_POINT('Ctrl Pts',(178.812916258969,2.22044604925031E-15,
38.45));
#19501=CARTESIAN_POINT('Ctrl Pts',(178.662665771103,0.00766025838161988,
38.4739453498545));
#19502=CARTESIAN_POINT('Ctrl Pts',(178.664312652589,0.00757270116505651,
38.4693721648001));
#19503=CARTESIAN_POINT('Ctrl Pts',(178.670768458182,0.00689135909653072,
38.4515513889253));
#19504=CARTESIAN_POINT('Ctrl Pts',(178.689811944466,0.00496920533963629,
38.3991254694919));
#19505=CARTESIAN_POINT('Ctrl Pts',(178.709764883196,0.00276026299996931,
38.3441919684076));
#19506=CARTESIAN_POINT('Ctrl Pts',(178.727201211343,0.00110274141105337,
38.2962200342644));
#19507=CARTESIAN_POINT('Ctrl Pts',(178.737862157161,0.000211760193833221,
38.2668827645598));
#19508=CARTESIAN_POINT('Ctrl Pts',(178.740836000832,1.66580200687153E-15,
38.2586896296938));
#19509=CARTESIAN_POINT('Ctrl Pts',(178.741944172646,1.66533453693773E-15,
38.2556349368385));
#19510=CARTESIAN_POINT('Ctrl Pts',(178.537807503284,0.0149175389192058,
38.4283524243692));
#19511=CARTESIAN_POINT('Ctrl Pts',(178.540562605001,0.0145270880491169,
38.4206441795725));
#19512=CARTESIAN_POINT('Ctrl Pts',(178.548129056013,0.0124870215921244,
38.3998601077916));
#19513=CARTESIAN_POINT('Ctrl Pts',(178.587627771362,0.00738392785094328,
38.2924874843148));
#19514=CARTESIAN_POINT('Ctrl Pts',(178.614538362218,0.00313671619344931,
38.2181107712228));
#19515=CARTESIAN_POINT('Ctrl Pts',(178.647624171299,0.00102987596989992,
38.1266989348736));
#19516=CARTESIAN_POINT('Ctrl Pts',(178.666537253803,0.000407918176736971,
38.0738320437369));
#19517=CARTESIAN_POINT('Ctrl Pts',(178.669110050143,1.11050312057989E-15,
38.0664089817677));
#19518=CARTESIAN_POINT('Ctrl Pts',(178.670972086323,1.11022302462515E-15,
38.061269873677));
#19519=CARTESIAN_POINT('Ctrl Pts',(178.412949235465,0.0221748194567917,
38.3827594988839));
#19520=CARTESIAN_POINT('Ctrl Pts',(178.416788815217,0.0212514804521959,
38.3719446039049));
#19521=CARTESIAN_POINT('Ctrl Pts',(178.428787456164,0.018059442750159,38.3379328437124));
#19522=CARTESIAN_POINT('Ctrl Pts',(178.479303492309,0.00868912423993776,
38.1971252772954));
#19523=CARTESIAN_POINT('Ctrl Pts',(178.520861801226,0.0033049704669746,
38.0831735428938));
#19524=CARTESIAN_POINT('Ctrl Pts',(178.565879979014,0.000430856897763508,
37.9603421260445));
#19525=CARTESIAN_POINT('Ctrl Pts',(178.592381442498,-1.56457495638545E-5,
37.8878951389657));
#19526=CARTESIAN_POINT('Ctrl Pts',(178.597384099455,5.55111512312573E-16,
37.8741283338417));
#19527=CARTESIAN_POINT('Ctrl Pts',(178.6,5.55111512312573E-16,37.8669048105155));
#19528=CARTESIAN_POINT('',(178.787524038921,0.00040297784403398,38.5195382753398));
#19529=CARTESIAN_POINT('Ctrl Pts',(178.812916258969,1.77635683940025E-15,
38.45));
#19530=CARTESIAN_POINT('Ctrl Pts',(178.812792389797,1.77661612872642E-15,
38.4503392180603));
#19531=CARTESIAN_POINT('Ctrl Pts',(178.812666912028,2.29080308876542E-8,
38.4506828414828));
#19532=CARTESIAN_POINT('Ctrl Pts',(178.812507168468,1.04590663241311E-7,
38.451120307067));
#19533=CARTESIAN_POINT('Ctrl Pts',(178.812339990782,1.90074632413641E-7,
38.4515781313736));
#19534=CARTESIAN_POINT('Ctrl Pts',(178.812135423681,3.38991576868653E-7,
38.4521383523834));
#19535=CARTESIAN_POINT('Ctrl Pts',(178.811876024071,6.76277157829475E-7,
38.4528487410224));
#19536=CARTESIAN_POINT('Ctrl Pts',(178.811582600925,1.05780200312327E-6,
38.4536523061046));
#19537=CARTESIAN_POINT('Ctrl Pts',(178.81121902708,1.68218510003301E-6,
38.454647990168));
#19538=CARTESIAN_POINT('Ctrl Pts',(178.81078427153,2.84078831658263E-6,
38.4558386172768));
#19539=CARTESIAN_POINT('Ctrl Pts',(178.810308592603,4.10845041919785E-6,
38.4571413176687));
#19540=CARTESIAN_POINT('Ctrl Pts',(178.809748146625,6.030430202368E-6,38.4586761668976));
#19541=CARTESIAN_POINT('Ctrl Pts',(178.809125174397,8.98260863735345E-6,
38.4603822551952));
#19542=CARTESIAN_POINT('Ctrl Pts',(178.808193484876,1.33977552344303E-5,
38.4629338048754));
#19543=CARTESIAN_POINT('Ctrl Pts',(178.807123623568,2.02240544095713E-5,
38.4658637622743));
#19544=CARTESIAN_POINT('Ctrl Pts',(178.806029976226,2.96381288054093E-5,
38.4688588617692));
#19545=CARTESIAN_POINT('Ctrl Pts',(178.805292443249,3.59867843904441E-5,
38.4708786944512));
#19546=CARTESIAN_POINT('Ctrl Pts',(178.804545203554,4.34635709253636E-5,
38.4729251106001));
#19547=CARTESIAN_POINT('Ctrl Pts',(178.803814942525,5.17716369792254E-5,
38.474925026849));
#19548=CARTESIAN_POINT('Ctrl Pts',(178.80317860389,5.90111625757292E-5,
38.4766677242206));
#19549=CARTESIAN_POINT('Ctrl Pts',(178.802555399229,6.6863151583119E-5,
38.4783744513132));
#19550=CARTESIAN_POINT('Ctrl Pts',(178.801949204039,7.51735349577842E-5,
38.4800345928624));
#19551=CARTESIAN_POINT('Ctrl Pts',(178.801382229325,8.29462413561495E-5,
38.481587324218));
#19552=CARTESIAN_POINT('Ctrl Pts',(178.800830323152,9.11060767190131E-5,
38.483098785948));
#19553=CARTESIAN_POINT('Ctrl Pts',(178.800280785453,9.97858253111161E-5,
38.4846037562484));
#19554=CARTESIAN_POINT('Ctrl Pts',(178.799730342786,0.000108479867530143,
38.4861112049022));
#19555=CARTESIAN_POINT('Ctrl Pts',(178.799179179204,0.000117743550685572,
38.4876206225174));
#19556=CARTESIAN_POINT('Ctrl Pts',(178.798613206839,0.000127862606367657,
38.4891705875312));
#19557=CARTESIAN_POINT('Ctrl Pts',(178.798000470497,0.000138817758135477,
38.4908486197997));
#19558=CARTESIAN_POINT('Ctrl Pts',(178.797370559065,0.000150785769506228,
38.4925736784058));
#19559=CARTESIAN_POINT('Ctrl Pts',(178.79672645219,0.000163820813490645,
38.4943376017011));
#19560=CARTESIAN_POINT('Ctrl Pts',(178.795973597268,0.000179056634472028,
38.4963993377092));
#19561=CARTESIAN_POINT('Ctrl Pts',(178.795201645712,0.000195768932648973,
38.4985133566153));
#19562=CARTESIAN_POINT('Ctrl Pts',(178.794439465589,0.00021337220547224,
38.50060060215));
#19563=CARTESIAN_POINT('Ctrl Pts',(178.793524503989,0.000234504111399393,
38.5031062428186));
#19564=CARTESIAN_POINT('Ctrl Pts',(178.792625243217,0.0002569141979263,
38.5055688657824));
#19565=CARTESIAN_POINT('Ctrl Pts',(178.791809195932,0.000278444418397861,
38.5078035940878));
#19566=CARTESIAN_POINT('Ctrl Pts',(178.791180207023,0.000295039375735335,
38.509526066969));
#19567=CARTESIAN_POINT('Ctrl Pts',(178.790601441912,0.000311061767359691,
38.5111109936911));
#19568=CARTESIAN_POINT('Ctrl Pts',(178.79009691346,0.000325452799612158,
38.5124926209708));
#19569=CARTESIAN_POINT('Ctrl Pts',(178.789638615777,0.000338525157990883,
38.5137476474782));
#19570=CARTESIAN_POINT('Ctrl Pts',(178.789241892366,0.000350230035308143,
38.5148340510745));
#19571=CARTESIAN_POINT('Ctrl Pts',(178.788911958311,0.000360129645157414,
38.5157375543241));
#19572=CARTESIAN_POINT('Ctrl Pts',(178.78860236805,0.00036941884325196,
38.516585347398));
#19573=CARTESIAN_POINT('Ctrl Pts',(178.788351785867,0.000377107969535637,
38.5172715489645));
#19574=CARTESIAN_POINT('Ctrl Pts',(178.788149176854,0.000383380392984911,
38.5178263793466));
#19575=CARTESIAN_POINT('Ctrl Pts',(178.787959584021,0.000389249858125049,
38.5183455658481));
#19576=CARTESIAN_POINT('Ctrl Pts',(178.787812084152,0.000393876622551518,
38.5187494837048));
#19577=CARTESIAN_POINT('Ctrl Pts',(178.787681864855,0.000397984058347234,
38.5191060801148));
#19578=CARTESIAN_POINT('Ctrl Pts',(178.787627357716,0.000399703347116144,
38.519255344092));
#19579=CARTESIAN_POINT('Ctrl Pts',(178.787575672948,0.000401338993554701,
38.519396879218));
#19580=CARTESIAN_POINT('Ctrl Pts',(178.787524038921,0.000402977844033536,
38.5195382753398));
#19581=CARTESIAN_POINT('Ctrl Pts',(178.412949235465,0.0221748194567917,
38.3827594988839));
#19582=CARTESIAN_POINT('Ctrl Pts',(178.537807503284,0.0149175389192058,
38.4283524243692));
#19583=CARTESIAN_POINT('Ctrl Pts',(178.662665771103,0.00766025838161988,
38.4739453498545));
#19584=CARTESIAN_POINT('Ctrl Pts',(178.787524038921,0.00040297784403398,
38.5195382753398));
#19585=CARTESIAN_POINT('Ctrl Pts',(178.412949235465,0.0221748194567911,
38.3827594988839));
#19586=CARTESIAN_POINT('Ctrl Pts',(178.240471017511,0.0636522405289915,
38.8685766805066));
#19587=CARTESIAN_POINT('Ctrl Pts',(178.066773051231,0.169426085453293,39.3947605243754));
#19588=CARTESIAN_POINT('Ctrl Pts',(177.858376073723,0.4624110846645,40.2928391623376));
#19589=CARTESIAN_POINT('Ctrl Pts',(177.799999999912,0.62257825368506,40.6717586072261));
#19590=CARTESIAN_POINT('Ctrl Pts',(177.8,0.800000000395797,41.0213168380085));
#19591=CARTESIAN_POINT('Ctrl Pts',(178.537807503284,0.0149175389192054,
38.4283524243692));
#19592=CARTESIAN_POINT('Ctrl Pts',(178.363766365304,0.0444484291304303,
38.9141666714197));
#19593=CARTESIAN_POINT('Ctrl Pts',(178.18361402036,0.137778888719998,39.439427238818));
#19594=CARTESIAN_POINT('Ctrl Pts',(177.955395603962,0.414097686712283,40.3338925283666));
#19595=CARTESIAN_POINT('Ctrl Pts',(177.885823288757,0.568803257711311,40.7106223452905));
#19596=CARTESIAN_POINT('Ctrl Pts',(177.872973082299,0.743827073473452,41.0573334705988));
#19597=CARTESIAN_POINT('Ctrl Pts',(178.662665771103,0.00766025838161969,
38.4739453498545));
#19598=CARTESIAN_POINT('Ctrl Pts',(178.486833473156,0.0252372669559836,
38.9597325112783));
#19599=CARTESIAN_POINT('Ctrl Pts',(178.300397971406,0.106138282654787,39.4840892505963));
#19600=CARTESIAN_POINT('Ctrl Pts',(178.05241766608,0.365784202340891,40.374947182902));
#19601=CARTESIAN_POINT('Ctrl Pts',(177.971553852029,0.515058096066276,40.7494851784996));
#19602=CARTESIAN_POINT('Ctrl Pts',(177.945946164598,0.687654146551106,41.0933501031891));
#19603=CARTESIAN_POINT('Ctrl Pts',(178.787524038921,0.00040297784403398,
38.5195382753398));
#19604=CARTESIAN_POINT('Ctrl Pts',(178.61012882095,0.00603345555742248,
39.0053225021914));
#19605=CARTESIAN_POINT('Ctrl Pts',(178.417238940535,0.0744910859214918,
39.528755965039));
#19606=CARTESIAN_POINT('Ctrl Pts',(178.149437196319,0.317470804388674,40.416000548931));
#19607=CARTESIAN_POINT('Ctrl Pts',(178.057377140874,0.461283100092528,40.7883489165639));
#19608=CARTESIAN_POINT('Ctrl Pts',(178.018919246896,0.631481219628761,41.1293667357794));
#19609=CARTESIAN_POINT('',(178.018919246896,0.631481219628701,41.1293667357793));
#19610=CARTESIAN_POINT('Ctrl Pts',(178.787524038921,0.00040297784403398,
38.5195382753398));
#19611=CARTESIAN_POINT('Ctrl Pts',(178.61012882095,0.00603345555742248,
39.0053225021914));
#19612=CARTESIAN_POINT('Ctrl Pts',(178.417238940535,0.0744910859214918,
39.528755965039));
#19613=CARTESIAN_POINT('Ctrl Pts',(178.149437196319,0.317470804388674,40.416000548931));
#19614=CARTESIAN_POINT('Ctrl Pts',(178.057377140874,0.461283100092528,40.7883489165639));
#19615=CARTESIAN_POINT('Ctrl Pts',(178.018919246896,0.631481219628761,41.1293667357794));
#19616=CARTESIAN_POINT('',(178.018919246896,0.631481219628701,41.1293667357793));
#19617=CARTESIAN_POINT('Origin',(177.9,6.00000000000001,38.45));
#19618=CARTESIAN_POINT('',(177.8,0.973333333333333,41.3435483791052));
#19619=CARTESIAN_POINT('',(178.,0.800000000000003,41.4433259094192));
#19620=CARTESIAN_POINT('',(177.8,0.973333333333333,41.3435483791052));
#19621=CARTESIAN_POINT('',(178.,3.00667409058085,43.65));
#19622=CARTESIAN_POINT('Origin',(178.,6.00000000000001,38.45));
#19623=CARTESIAN_POINT('',(177.8,3.10645162089482,43.4766666666667));
#19624=CARTESIAN_POINT('',(178.,3.00667409058085,43.65));
#19625=CARTESIAN_POINT('Origin',(177.8,6.00000000000001,38.45));
#19626=CARTESIAN_POINT('Ctrl Pts',(177.8,0.800000000395732,41.0213168380084));
#19627=CARTESIAN_POINT('Ctrl Pts',(177.8,0.85616853425096,41.1319806866355));
#19628=CARTESIAN_POINT('Ctrl Pts',(177.8,0.913326151321778,41.2393040181827));
#19629=CARTESIAN_POINT('Ctrl Pts',(177.8,0.973333333333334,41.3435483791052));
#19630=CARTESIAN_POINT('Ctrl Pts',(177.872973082299,0.743827073473389,41.0573334705987));
#19631=CARTESIAN_POINT('Ctrl Pts',(177.868914723125,0.799233317184012,41.1670960723289));
#19632=CARTESIAN_POINT('Ctrl Pts',(177.866666666667,0.856146146238369,41.2736016445264));
#19633=CARTESIAN_POINT('Ctrl Pts',(177.866666666667,0.915555555555557,41.3768075558765));
#19634=CARTESIAN_POINT('Ctrl Pts',(177.945946164598,0.687654146551045,41.093350103189));
#19635=CARTESIAN_POINT('Ctrl Pts',(177.937829446251,0.742298100117064,41.2022114580222));
#19636=CARTESIAN_POINT('Ctrl Pts',(177.933333333333,0.79896614115496,41.3078992708702));
#19637=CARTESIAN_POINT('Ctrl Pts',(177.933333333333,0.857777777777779,41.4100667326478));
#19638=CARTESIAN_POINT('Ctrl Pts',(178.018919246896,0.631481219628701,41.1293667357793));
#19639=CARTESIAN_POINT('Ctrl Pts',(178.006744169376,0.685362883050116,41.2373268437155));
#19640=CARTESIAN_POINT('Ctrl Pts',(178.,0.74178613607155,41.3421968972139));
#19641=CARTESIAN_POINT('Ctrl Pts',(178.,0.800000000000002,41.4433259094191));
#19642=CARTESIAN_POINT('Ctrl Pts',(177.8,0.973333333333334,41.3435483791052));
#19643=CARTESIAN_POINT('Ctrl Pts',(177.8,0.913326151321778,41.2393040181827));
#19644=CARTESIAN_POINT('Ctrl Pts',(177.8,0.85616853425096,41.1319806866355));
#19645=CARTESIAN_POINT('Ctrl Pts',(177.8,0.800000000395732,41.0213168380084));
#19646=CARTESIAN_POINT('Ctrl Pts',(178.018919246896,0.631481219628701,41.1293667357793));
#19647=CARTESIAN_POINT('Ctrl Pts',(178.006744169376,0.685362883050116,41.2373268437155));
#19648=CARTESIAN_POINT('Ctrl Pts',(178.,0.74178613607155,41.3421968972139));
#19649=CARTESIAN_POINT('Ctrl Pts',(178.,0.800000000000002,41.4433259094191));
#19650=CARTESIAN_POINT('Ctrl Pts',(177.8,3.42868316060635,43.6499999989011));
#19651=CARTESIAN_POINT('Ctrl Pts',(177.799999999778,3.74718302197855,43.8116577622765));
#19652=CARTESIAN_POINT('Ctrl Pts',(177.852262520974,4.10069604234112,43.9610343215402));
#19653=CARTESIAN_POINT('Ctrl Pts',(178.027580341374,4.92462867457202,44.2486946146566));
#19654=CARTESIAN_POINT('Ctrl Pts',(178.227442457241,5.54472605716147,44.3832148024821));
#19655=CARTESIAN_POINT('Ctrl Pts',(178.412949792571,6.06724207026202,44.4278253145154));
#19656=CARTESIAN_POINT('Ctrl Pts',(177.872973082248,3.39266652802731,43.706172925833));
#19657=CARTESIAN_POINT('Ctrl Pts',(177.884801501945,3.70854266993171,43.8657195742618));
#19658=CARTESIAN_POINT('Ctrl Pts',(177.94736184287,4.0600303778348,44.0100109505439));
#19659=CARTESIAN_POINT('Ctrl Pts',(178.14244940435,4.88027329102046,44.2832673714004));
#19660=CARTESIAN_POINT('Ctrl Pts',(178.350875881265,5.49908229532861,44.4034058024122));
#19661=CARTESIAN_POINT('Ctrl Pts',(178.537808064946,6.02164914272028,44.4350825564341));
#19662=CARTESIAN_POINT('Ctrl Pts',(177.945946164496,3.35664989544827,43.7623458527649));
#19663=CARTESIAN_POINT('Ctrl Pts',(177.969158641282,3.66999188322933,43.9195329256993));
#19664=CARTESIAN_POINT('Ctrl Pts',(178.042561961955,4.0193437759176,44.0590539599822));
#19665=CARTESIAN_POINT('Ctrl Pts',(178.257082225015,4.83596655149052,44.317714473429));
#19666=CARTESIAN_POINT('Ctrl Pts',(178.473297911834,5.45363322129503,44.4233504482635));
#19667=CARTESIAN_POINT('Ctrl Pts',(178.662666337321,5.97605621517853,44.4423397983527));
#19668=CARTESIAN_POINT('Ctrl Pts',(178.018919246744,3.32063326286924,43.8185187796968));
#19669=CARTESIAN_POINT('Ctrl Pts',(178.053960143449,3.63135153118249,43.9735947376847));
#19670=CARTESIAN_POINT('Ctrl Pts',(178.137661283851,3.97867811141129,44.1080305889859));
#19671=CARTESIAN_POINT('Ctrl Pts',(178.37195128799,4.79161116793896,44.3522872301728));
#19672=CARTESIAN_POINT('Ctrl Pts',(178.596731335858,5.40798945946218,44.4435414481936));
#19673=CARTESIAN_POINT('Ctrl Pts',(178.787524609695,5.93046328763679,44.4495970402714));
#19674=CARTESIAN_POINT('',(177.8,3.42868316035968,43.649999999388));
#19675=CARTESIAN_POINT('Ctrl Pts',(178.412949792571,6.06724207026202,44.4278253145154));
#19676=CARTESIAN_POINT('Ctrl Pts',(178.227442457241,5.54472605716147,44.3832148024821));
#19677=CARTESIAN_POINT('Ctrl Pts',(178.027580341374,4.92462867457202,44.2486946146566));
#19678=CARTESIAN_POINT('Ctrl Pts',(177.852262520974,4.10069604234112,43.9610343215402));
#19679=CARTESIAN_POINT('Ctrl Pts',(177.799999999778,3.74718302197855,43.8116577622765));
#19680=CARTESIAN_POINT('Ctrl Pts',(177.8,3.42868316060635,43.6499999989011));
#19681=CARTESIAN_POINT('',(178.018919246744,3.32063326286958,43.818518779697));
#19682=CARTESIAN_POINT('',(177.8,3.42868316035968,43.649999999388));
#19683=CARTESIAN_POINT('Ctrl Pts',(178.018919246744,3.32063326286924,43.8185187796968));
#19684=CARTESIAN_POINT('Ctrl Pts',(178.053960143449,3.63135153118249,43.9735947376847));
#19685=CARTESIAN_POINT('Ctrl Pts',(178.137661283851,3.97867811141129,44.1080305889859));
#19686=CARTESIAN_POINT('Ctrl Pts',(178.37195128799,4.79161116793896,44.3522872301728));
#19687=CARTESIAN_POINT('Ctrl Pts',(178.596731335858,5.40798945946218,44.4435414481936));
#19688=CARTESIAN_POINT('Ctrl Pts',(178.787524609695,5.93046328763679,44.4495970402714));
#19689=CARTESIAN_POINT('Ctrl Pts',(177.8,3.10645162089482,43.4766666666667));
#19690=CARTESIAN_POINT('Ctrl Pts',(177.8,3.20794511515403,43.5350903408981));
#19691=CARTESIAN_POINT('Ctrl Pts',(177.8,3.31591505255455,43.5927634272858));
#19692=CARTESIAN_POINT('Ctrl Pts',(177.8,3.42868316060669,43.6499999989013));
#19693=CARTESIAN_POINT('Ctrl Pts',(177.866666666667,3.0731924441235,43.5344444444444));
#19694=CARTESIAN_POINT('Ctrl Pts',(177.866666666667,3.17367489207974,43.5922861203885));
#19695=CARTESIAN_POINT('Ctrl Pts',(177.86883755389,3.28081680397103,43.6497131392107));
#19696=CARTESIAN_POINT('Ctrl Pts',(177.872973082248,3.39266652802765,43.7061729258332));
#19697=CARTESIAN_POINT('Ctrl Pts',(177.933333333333,3.03993326735218,43.5922222222222));
#19698=CARTESIAN_POINT('Ctrl Pts',(177.933333333333,3.13940466900545,43.649481899879));
#19699=CARTESIAN_POINT('Ctrl Pts',(177.93767510778,3.24571855538751,43.7066628511355));
#19700=CARTESIAN_POINT('Ctrl Pts',(177.945946164496,3.35664989544862,43.7623458527651));
#19701=CARTESIAN_POINT('Ctrl Pts',(178.,3.00667409058085,43.65));
#19702=CARTESIAN_POINT('Ctrl Pts',(178.,3.10513444593116,43.7066776793694));
#19703=CARTESIAN_POINT('Ctrl Pts',(178.00651266167,3.21062030680399,43.7636125630604));
#19704=CARTESIAN_POINT('Ctrl Pts',(178.018919246744,3.32063326286958,43.818518779697));
#19705=CARTESIAN_POINT('Ctrl Pts',(177.8,3.42868316060669,43.6499999989013));
#19706=CARTESIAN_POINT('Ctrl Pts',(177.8,3.31591505255455,43.5927634272858));
#19707=CARTESIAN_POINT('Ctrl Pts',(177.8,3.20794511515403,43.5350903408981));
#19708=CARTESIAN_POINT('Ctrl Pts',(177.8,3.10645162089482,43.4766666666667));
#19709=CARTESIAN_POINT('Ctrl Pts',(178.,3.00667409058085,43.65));
#19710=CARTESIAN_POINT('Ctrl Pts',(178.,3.10513444593116,43.7066776793694));
#19711=CARTESIAN_POINT('Ctrl Pts',(178.00651266167,3.21062030680399,43.7636125630604));
#19712=CARTESIAN_POINT('Ctrl Pts',(178.018919246744,3.32063326286958,43.818518779697));
#19713=CARTESIAN_POINT('Origin',(177.8,63.5,-31.75));
#19714=CARTESIAN_POINT('',(177.8,123.993325909419,43.65));
#19715=CARTESIAN_POINT('',(177.8,92.25,43.65));
#19716=CARTESIAN_POINT('',(177.8,126.2,41.4433259094192));
#19717=CARTESIAN_POINT('Origin',(177.8,121.,38.45));
#19718=CARTESIAN_POINT('',(177.8,126.2,-104.943325909419));
#19719=CARTESIAN_POINT('',(177.8,126.2,-66.85));
#19720=CARTESIAN_POINT('',(177.8,123.993325909419,-107.15));
#19721=CARTESIAN_POINT('Origin',(177.8,121.,-101.95));
#19722=CARTESIAN_POINT('',(177.8,34.75,-107.15));
#19723=CARTESIAN_POINT('Ctrl Pts',(181.949550208499,0.0221746857420428,
38.3827579327069));
#19724=CARTESIAN_POINT('Ctrl Pts',(181.93931132845,0.0197124559678562,38.3539182157356));
#19725=CARTESIAN_POINT('Ctrl Pts',(181.84754199691,-0.000377263094500332,
38.0974645231953));
#19726=CARTESIAN_POINT('Ctrl Pts',(181.77034781043,2.07279408068869E-16,
37.8885753052303));
#19727=CARTESIAN_POINT('Ctrl Pts',(181.7625,5.55111512312556E-16,37.8669048105155));
#19728=CARTESIAN_POINT('Ctrl Pts',(181.824691935409,0.0149174437260072,
38.4283508582629));
#19729=CARTESIAN_POINT('Ctrl Pts',(181.817345007617,0.013876249080669,38.4077955695789));
#19730=CARTESIAN_POINT('Ctrl Pts',(181.752629283213,-0.00242179847811128,
38.2259457666522));
#19731=CARTESIAN_POINT('Ctrl Pts',(181.69711408673,8.79071517678641E-16,
38.076687125913));
#19732=CARTESIAN_POINT('Ctrl Pts',(181.691527913677,1.11022302462513E-15,
38.061269873677));
#19733=CARTESIAN_POINT('Ctrl Pts',(181.69983366232,0.00766020170997153,
38.4739437838189));
#19734=CARTESIAN_POINT('Ctrl Pts',(181.695441999281,0.00742672173854637,
38.4617486824133));
#19735=CARTESIAN_POINT('Ctrl Pts',(181.655779237654,0.00233129106079364,
38.3525367447957));
#19736=CARTESIAN_POINT('Ctrl Pts',(181.62388036303,1.55087664284178E-15,
38.2647989465957));
#19737=CARTESIAN_POINT('Ctrl Pts',(181.620555827354,1.66533453693771E-15,
38.2556349368385));
#19738=CARTESIAN_POINT('Ctrl Pts',(181.57497538923,0.000402959693935889,
38.5195367093749));
#19739=CARTESIAN_POINT('Ctrl Pts',(181.573558278095,0.000357981970936656,
38.5156560509973));
#19740=CARTESIAN_POINT('Ctrl Pts',(181.560928464961,-7.92708613026129E-6,
38.481069555198));
#19741=CARTESIAN_POINT('Ctrl Pts',(181.550646639331,2.22267096288126E-15,
38.4529107672783));
#19742=CARTESIAN_POINT('Ctrl Pts',(181.549583741031,2.22044604925029E-15,
38.45));
#19743=CARTESIAN_POINT('',(181.949550208499,0.0221746857420428,38.3827579327069));
#19744=CARTESIAN_POINT('Ctrl Pts',(181.7625,4.44089209850063E-16,37.8669048105155));
#19745=CARTESIAN_POINT('Ctrl Pts',(181.76304148203,4.20005004317793E-16,
37.8684000280116));
#19746=CARTESIAN_POINT('Ctrl Pts',(181.763584479695,5.09304599544949E-7,
37.8698993823924));
#19747=CARTESIAN_POINT('Ctrl Pts',(181.764185485109,1.77553950320153E-6,
37.8715567677798));
#19748=CARTESIAN_POINT('Ctrl Pts',(181.764814435413,3.10065040867961E-6,
37.8732912164553));
#19749=CARTESIAN_POINT('Ctrl Pts',(181.765506905312,5.25009810737027E-6,
37.8751987104973));
#19750=CARTESIAN_POINT('Ctrl Pts',(181.766307739637,9.06185204052612E-6,
37.8774013223017));
#19751=CARTESIAN_POINT('Ctrl Pts',(181.767138138677,1.30143259816557E-5,
37.879685248786));
#19752=CARTESIAN_POINT('Ctrl Pts',(181.768084982826,1.87485342410978E-5,
37.882286296731));
#19753=CARTESIAN_POINT('Ctrl Pts',(181.769177981748,2.78726356962578E-5,
37.8852852358398));
#19754=CARTESIAN_POINT('Ctrl Pts',(181.770320300149,3.74084447238513E-5,
37.8884194963221));
#19755=CARTESIAN_POINT('Ctrl Pts',(181.771622177173,5.06509191333375E-5,
37.8919881335616));
#19756=CARTESIAN_POINT('Ctrl Pts',(181.773096907529,7.01871096291384E-5,
37.896027172726));
#19757=CARTESIAN_POINT('Ctrl Pts',(181.774657138679,9.08559545094126E-5,
37.9003003842292));
#19758=CARTESIAN_POINT('Ctrl Pts',(181.776410738128,0.000118594684243597,
37.9050998197267));
#19759=CARTESIAN_POINT('Ctrl Pts',(181.778352315947,0.000157075370967652,
37.9104106590806));
#19760=CARTESIAN_POINT('Ctrl Pts',(181.780451023138,0.000198670249723156,
37.9161512977704));
#19761=CARTESIAN_POINT('Ctrl Pts',(181.782769206869,0.000252878342011502,
37.9224890235653));
#19762=CARTESIAN_POINT('Ctrl Pts',(181.785278039374,0.000324340171413695,
37.9293453635552));
#19763=CARTESIAN_POINT('Ctrl Pts',(181.788122975606,0.000405375612125061,
37.937120234943));
#19764=CARTESIAN_POINT('Ctrl Pts',(181.791212773971,0.000508738325902519,
37.9455611859274));
#19765=CARTESIAN_POINT('Ctrl Pts',(181.794481379312,0.000639510998152626,
37.9544887994803));
#19766=CARTESIAN_POINT('Ctrl Pts',(181.799555799721,0.000842531995694803,
37.9683486753855));
#19767=CARTESIAN_POINT('Ctrl Pts',(181.805059381922,0.00111289751450502,
37.9833765823867));
#19768=CARTESIAN_POINT('Ctrl Pts',(181.810697440792,0.00145319066376182,
37.998773281532));
#19769=CARTESIAN_POINT('Ctrl Pts',(181.814293586,0.00167024117814912,38.0085938185504));
#19770=CARTESIAN_POINT('Ctrl Pts',(181.817943390686,0.00191521782814626,
38.0185615609443));
#19771=CARTESIAN_POINT('Ctrl Pts',(181.821578859223,0.0021844270804634,
38.0284922998829));
#19772=CARTESIAN_POINT('Ctrl Pts',(181.824987110976,0.00243681075451073,
38.0378023676378));
#19773=CARTESIAN_POINT('Ctrl Pts',(181.828382262706,0.00271034782317473,
38.0470785394244));
#19774=CARTESIAN_POINT('Ctrl Pts',(181.831725566481,0.00300073968331871,
38.0562161880863));
#19775=CARTESIAN_POINT('Ctrl Pts',(181.834646587955,0.0032544530508039,
38.0641996887662));
#19776=CARTESIAN_POINT('Ctrl Pts',(181.837528033025,0.0035209403924873,
38.072077438301));
#19777=CARTESIAN_POINT('Ctrl Pts',(181.84036024516,0.00379790114339729,
38.0798239992515));
#19778=CARTESIAN_POINT('Ctrl Pts',(181.843021786712,0.00405817209476014,
38.0871037483919));
#19779=CARTESIAN_POINT('Ctrl Pts',(181.84563977042,0.00432762707091396,
38.0942674097725));
#19780=CARTESIAN_POINT('Ctrl Pts',(181.848222212492,0.00460594527901903,
38.1013379934289));
#19781=CARTESIAN_POINT('Ctrl Pts',(181.850701024556,0.00487309494308377,
38.1081248438525));
#19782=CARTESIAN_POINT('Ctrl Pts',(181.853147008996,0.00514835430903795,
38.1148256972557));
#19783=CARTESIAN_POINT('Ctrl Pts',(181.855583689387,0.00543381221564498,
38.1215063521776));
#19784=CARTESIAN_POINT('Ctrl Pts',(181.858071001312,0.00572520162318504,
38.1283258237515));
#19785=CARTESIAN_POINT('Ctrl Pts',(181.860551411675,0.00602752312911085,
38.1351319692169));
#19786=CARTESIAN_POINT('Ctrl Pts',(181.863055940733,0.00634484643309796,
38.1420115697532));
#19787=CARTESIAN_POINT('Ctrl Pts',(181.865640315095,0.0066722861202117,
38.1491104944738));
#19788=CARTESIAN_POINT('Ctrl Pts',(181.868250295974,0.00701574757250298,
38.1562874412164));
#19789=CARTESIAN_POINT('Ctrl Pts',(181.870899527483,0.00737805831443783,
38.1635813068402));
#19790=CARTESIAN_POINT('Ctrl Pts',(181.873695982834,0.00776050349121822,
38.1712805092238));
#19791=CARTESIAN_POINT('Ctrl Pts',(181.876536050774,0.00816400147160706,
38.1791096716376));
#19792=CARTESIAN_POINT('Ctrl Pts',(181.879415035157,0.00858931359615633,
38.1870569678962));
#19793=CARTESIAN_POINT('Ctrl Pts',(181.882513643039,0.00904707068189298,
38.1956105241314));
#19794=CARTESIAN_POINT('Ctrl Pts',(181.885657154427,0.00953016157912426,
38.2043004729611));
#19795=CARTESIAN_POINT('Ctrl Pts',(181.888818575754,0.0100356859835848,
38.2130529045922));
#19796=CARTESIAN_POINT('Ctrl Pts',(181.892379707013,0.0106051256667839,
38.2229119378085));
#19797=CARTESIAN_POINT('Ctrl Pts',(181.895963258973,0.0112031276223819,
38.2328494834971));
#19798=CARTESIAN_POINT('Ctrl Pts',(181.899508342925,0.0118193646321622,
38.2426964227595));
#19799=CARTESIAN_POINT('Ctrl Pts',(181.906183227132,0.0129796504642326,
38.2612367959178));
#19800=CARTESIAN_POINT('Ctrl Pts',(181.912718758197,0.0142069749798927,
38.2794495139526));
#19801=CARTESIAN_POINT('Ctrl Pts',(181.918632200457,0.0153837014308582,
38.2959720321497));
#19802=CARTESIAN_POINT('Ctrl Pts',(181.921657512848,0.0159857137540303,
38.3044249394131));
#19803=CARTESIAN_POINT('Ctrl Pts',(181.924519594541,0.0165735780399693,
38.3124338071031));
#19804=CARTESIAN_POINT('Ctrl Pts',(181.927164975675,0.0171299943247164,
38.3198448741925));
#19805=CARTESIAN_POINT('Ctrl Pts',(181.929548820379,0.0176314003402352,
38.3265232438267));
#19806=CARTESIAN_POINT('Ctrl Pts',(181.931756490456,0.0181071304378864,
38.3327155370088));
#19807=CARTESIAN_POINT('Ctrl Pts',(181.933762899352,0.0185468540560407,
38.3383480472888));
#19808=CARTESIAN_POINT('Ctrl Pts',(181.935639369544,0.0189581003699228,
38.3436157859203));
#19809=CARTESIAN_POINT('Ctrl Pts',(181.937339669048,0.0193377715846431,
38.3483934857085));
#19810=CARTESIAN_POINT('Ctrl Pts',(181.93885852085,0.0196810446211592,38.3526637724704));
#19811=CARTESIAN_POINT('Ctrl Pts',(181.940271287443,0.0200003415252573,
38.3566357982273));
#19812=CARTESIAN_POINT('Ctrl Pts',(181.941527033176,0.0202881189884772,
38.3601687015716));
#19813=CARTESIAN_POINT('Ctrl Pts',(181.942636217166,0.0205444571591845,
38.3632902746199));
#19814=CARTESIAN_POINT('Ctrl Pts',(181.943711761215,0.0207930209653079,
38.3663171748893));
#19815=CARTESIAN_POINT('Ctrl Pts',(181.94464940078,0.0210119940283042,38.3689570326758));
#19816=CARTESIAN_POINT('Ctrl Pts',(181.945474089021,0.021205750697401,38.3712791369017));
#19817=CARTESIAN_POINT('Ctrl Pts',(181.946277108126,0.0213944163034733,
38.3735402265622));
#19818=CARTESIAN_POINT('Ctrl Pts',(181.946972949247,0.021559156053933,38.3754998027936));
#19819=CARTESIAN_POINT('Ctrl Pts',(181.947600825471,0.0217084836580261,
38.3772679633097));
#19820=CARTESIAN_POINT('Ctrl Pts',(181.948209078132,0.0218531441962382,
38.3789808619627));
#19821=CARTESIAN_POINT('Ctrl Pts',(181.94875350008,0.0219833332935568,38.3805139890893));
#19822=CARTESIAN_POINT('Ctrl Pts',(181.949286053238,0.0221112095448139,
38.3820139178392));
#19823=CARTESIAN_POINT('Ctrl Pts',(181.949374298298,0.0221323988802871,
38.3822624588557));
#19824=CARTESIAN_POINT('Ctrl Pts',(181.949462255764,0.022153535006527,38.3825101974093));
#19825=CARTESIAN_POINT('Ctrl Pts',(181.949550208499,0.0221746857420413,
38.3827579327069));
#19826=CARTESIAN_POINT('',(181.57497538923,0.000402959693935889,38.5195367093749));
#19827=CARTESIAN_POINT('Ctrl Pts',(181.57497538923,0.000402959693935889,
38.5195367093749));
#19828=CARTESIAN_POINT('Ctrl Pts',(181.69983366232,0.00766020170997153,
38.4739437838189));
#19829=CARTESIAN_POINT('Ctrl Pts',(181.824691935409,0.0149174437260072,
38.4283508582629));
#19830=CARTESIAN_POINT('Ctrl Pts',(181.949550208499,0.0221746857420428,
38.3827579327069));
#19831=CARTESIAN_POINT('Ctrl Pts',(181.57497538923,0.000402959693936111,
38.5195367093749));
#19832=CARTESIAN_POINT('Ctrl Pts',(181.574851529658,0.00039902851210055,
38.519197528716));
#19833=CARTESIAN_POINT('Ctrl Pts',(181.574726061451,0.000395069178890136,
38.5188539427319));
#19834=CARTESIAN_POINT('Ctrl Pts',(181.574566326858,0.000390081041366841,
38.518416520908));
#19835=CARTESIAN_POINT('Ctrl Pts',(181.574399158571,0.000384860766966021,
38.5179587424408));
#19836=CARTESIAN_POINT('Ctrl Pts',(181.574194600227,0.000378517204501205,
38.5173985742044));
#19837=CARTESIAN_POINT('Ctrl Pts',(181.573935208538,0.000370621645222613,
38.5166882477071));
#19838=CARTESIAN_POINT('Ctrl Pts',(181.573641794121,0.000361690476534324,
38.5158847522804));
#19839=CARTESIAN_POINT('Ctrl Pts',(181.573278227823,0.000350775602826365,
38.5148891495373));
#19840=CARTESIAN_POINT('Ctrl Pts',(181.572843478859,0.000338135634860848,
38.5136986128781));
#19841=CARTESIAN_POINT('Ctrl Pts',(181.572367805852,0.000324305834040387,
38.5123960079261));
#19842=CARTESIAN_POINT('Ctrl Pts',(181.571807364196,0.000308439823463236,
38.5108612635613));
#19843=CARTESIAN_POINT('Ctrl Pts',(181.571184395662,0.000291619369626517,
38.5091552820435));
#19844=CARTESIAN_POINT('Ctrl Pts',(181.570252722647,0.000266463744452544,
38.5066039221317));
#19845=CARTESIAN_POINT('Ctrl Pts',(181.569182879842,0.000239333604321804,
38.503674166543));
#19846=CARTESIAN_POINT('Ctrl Pts',(181.568089252669,0.000214035990966366,
38.5006792470363));
#19847=CARTESIAN_POINT('Ctrl Pts',(181.567351730344,0.000196975739463386,
38.4986595276542));
#19848=CARTESIAN_POINT('Ctrl Pts',(181.566604501957,0.000180735411225578,
38.4966132148558));
#19849=CARTESIAN_POINT('Ctrl Pts',(181.565874252981,0.000165865156090739,
38.4946133876972));
#19850=CARTESIAN_POINT('Ctrl Pts',(181.565237923904,0.000152907416969221,
38.49287076537));
#19851=CARTESIAN_POINT('Ctrl Pts',(181.564614729409,0.00014097893488106,
38.4911641027617));
#19852=CARTESIAN_POINT('Ctrl Pts',(181.564008544896,0.000130048672500216,
38.4895040144456));
#19853=CARTESIAN_POINT('Ctrl Pts',(181.563441576379,0.00011982552339432,
38.487951322498));
#19854=CARTESIAN_POINT('Ctrl Pts',(181.562889677075,0.000110467742542563,
38.4864398910591));
#19855=CARTESIAN_POINT('Ctrl Pts',(181.562340146278,0.000101705034171395,
38.4849349404768));
#19856=CARTESIAN_POINT('Ctrl Pts',(181.561789713655,9.2927945483311E-5,
38.4834275201481));
#19857=CARTESIAN_POINT('Ctrl Pts',(181.561238560062,8.46975944274953E-5,
38.4819181200221));
#19858=CARTESIAN_POINT('Ctrl Pts',(181.56067259846,7.68526057823848E-5,
38.4803681636429));
#19859=CARTESIAN_POINT('Ctrl Pts',(181.560059870002,6.83593656547746E-5,
38.4786901304027));
#19860=CARTESIAN_POINT('Ctrl Pts',(181.559429967136,6.03338773008794E-5,
38.4769650596898));
#19861=CARTESIAN_POINT('Ctrl Pts',(181.558785869966,5.29249154554989E-5,
38.4752011147451));
#19862=CARTESIAN_POINT('Ctrl Pts',(181.558033019287,4.42649768435077E-5,
38.4731393339917));
#19863=CARTESIAN_POINT('Ctrl Pts',(181.557261073166,3.64754843892193E-5,
38.471025256065));
#19864=CARTESIAN_POINT('Ctrl Pts',(181.556498900774,2.98872215322987E-5,
38.4689379451134));
#19865=CARTESIAN_POINT('Ctrl Pts',(181.555583979329,2.19785869096659E-5,
38.4664323104691));
#19866=CARTESIAN_POINT('Ctrl Pts',(181.554684761097,1.58465131801333E-5,
38.4639696816724));
#19867=CARTESIAN_POINT('Ctrl Pts',(181.553868752768,1.14757415285993E-5,
38.4617349378622));
#19868=CARTESIAN_POINT('Ctrl Pts',(181.553239785674,8.10681568953756E-6,
38.4600124305416));
#19869=CARTESIAN_POINT('Ctrl Pts',(181.552661041472,5.75943763824285E-6,
38.4584274674403));
#19870=CARTESIAN_POINT('Ctrl Pts',(181.552156531242,4.1369507819411E-6,
38.4570458067133));
#19871=CARTESIAN_POINT('Ctrl Pts',(181.551698249181,2.66313206549139E-6,
38.4557907472771));
#19872=CARTESIAN_POINT('Ctrl Pts',(181.551301539411,1.77618418147096E-6,
38.4547043140198));
#19873=CARTESIAN_POINT('Ctrl Pts',(181.550971615919,1.20383124357915E-6,
38.4538007858999));
#19874=CARTESIAN_POINT('Ctrl Pts',(181.550662035304,6.66769231341577E-7,
38.4529529687611));
#19875=CARTESIAN_POINT('Ctrl Pts',(181.550411460152,4.02524086533268E-7,
38.4522667477014));
#19876=CARTESIAN_POINT('Ctrl Pts',(181.550208854898,2.44216733058522E-7,
38.4517118997389));
#19877=CARTESIAN_POINT('Ctrl Pts',(181.550019265284,9.60792622203152E-8,
38.4511926959744));
#19878=CARTESIAN_POINT('Ctrl Pts',(181.549871765901,4.12476565666961E-8,
38.4507887629029));
#19879=CARTESIAN_POINT('Ctrl Pts',(181.549741543983,1.55625716757868E-8,
38.4504321467835));
#19880=CARTESIAN_POINT('Ctrl Pts',(181.549687045568,4.81325671682278E-9,
38.4502829014529));
#19881=CARTESIAN_POINT('Ctrl Pts',(181.549635367948,1.77646490753008E-15,
38.4501413812976));
#19882=CARTESIAN_POINT('Ctrl Pts',(181.549583741031,1.77635683940025E-15,
38.45));
#19883=CARTESIAN_POINT('Ctrl Pts',(181.574975961468,5.93046172357687,44.4495970221434));
#19884=CARTESIAN_POINT('Ctrl Pts',(181.574444532932,5.93191700291845,44.4496138895458));
#19885=CARTESIAN_POINT('Ctrl Pts',(181.572770787455,5.93650035880571,44.449672474836));
#19886=CARTESIAN_POINT('Ctrl Pts',(181.565836964823,5.95548859185619,44.449843301418));
#19887=CARTESIAN_POINT('Ctrl Pts',(181.560226126263,5.97085451379058,44.4499402615516));
#19888=CARTESIAN_POINT('Ctrl Pts',(181.554178821344,5.98741591022133,44.449992182184));
#19889=CARTESIAN_POINT('Ctrl Pts',(181.55061386901,5.99717895300097,44.4500002913724));
#19890=CARTESIAN_POINT('Ctrl Pts',(181.549938048485,5.9990297223651,44.45));
#19891=CARTESIAN_POINT('Ctrl Pts',(181.549583741031,6.,44.45));
#19892=CARTESIAN_POINT('Ctrl Pts',(181.699834229027,5.97605464978202,44.4423397416411));
#19893=CARTESIAN_POINT('Ctrl Pts',(181.698187347511,5.9806278348658,44.4424272990258));
#19894=CARTESIAN_POINT('Ctrl Pts',(181.691731181696,5.99844959657613,44.4431086533954));
#19895=CARTESIAN_POINT('Ctrl Pts',(181.672687746495,6.05087537581987,44.4450308050866));
#19896=CARTESIAN_POINT('Ctrl Pts',(181.652734774536,6.10580896795632,44.447239748624));
#19897=CARTESIAN_POINT('Ctrl Pts',(181.635298667028,6.15378029848288,44.4488972633241));
#19898=CARTESIAN_POINT('Ctrl Pts',(181.624637758958,6.18311746495192,44.4497882438633));
#19899=CARTESIAN_POINT('Ctrl Pts',(181.62166399917,6.19131037030118,44.45));
#19900=CARTESIAN_POINT('Ctrl Pts',(181.620555827354,6.1943650631615,44.45));
#19901=CARTESIAN_POINT('Ctrl Pts',(181.824692496587,6.02164757598718,44.4350824611388));
#19902=CARTESIAN_POINT('Ctrl Pts',(181.821937394915,6.02935582072027,44.4354729132427));
#19903=CARTESIAN_POINT('Ctrl Pts',(181.814368169928,6.0501471994832,44.4375133635835));
#19904=CARTESIAN_POINT('Ctrl Pts',(181.774869846903,6.15751878131652,44.4426163977142));
#19905=CARTESIAN_POINT('Ctrl Pts',(181.747959001421,6.23189616960441,44.4468636541891));
#19906=CARTESIAN_POINT('Ctrl Pts',(181.714874888603,6.32330353191465,44.4489702868513));
#19907=CARTESIAN_POINT('Ctrl Pts',(181.69596209178,6.37616965773883,44.4495922345424));
#19908=CARTESIAN_POINT('Ctrl Pts',(181.693389949855,6.38359101823726,44.45));
#19909=CARTESIAN_POINT('Ctrl Pts',(181.691527913677,6.388730126323,44.45));
#19910=CARTESIAN_POINT('Ctrl Pts',(181.949550764146,6.06724050219233,44.4278251806365));
#19911=CARTESIAN_POINT('Ctrl Pts',(181.945711184342,6.07805539712614,44.4287485196519));
#19912=CARTESIAN_POINT('Ctrl Pts',(181.933709998201,6.11207446414045,44.4319413603754));
#19913=CARTESIAN_POINT('Ctrl Pts',(181.883194320107,6.25288098876544,44.4413115590186));
#19914=CARTESIAN_POINT('Ctrl Pts',(181.841635780004,6.36683339813076,44.4466958050519));
#19915=CARTESIAN_POINT('Ctrl Pts',(181.79661916996,6.4896603408434,44.4495694591275));
#19916=CARTESIAN_POINT('Ctrl Pts',(181.770117979333,6.56210656250854,44.4500159173546));
#19917=CARTESIAN_POINT('Ctrl Pts',(181.76511590054,6.57587166617334,44.45));
#19918=CARTESIAN_POINT('Ctrl Pts',(181.7625,6.5830951894845,44.45));
#19919=CARTESIAN_POINT('',(181.549583741031,6.,44.45));
#19920=CARTESIAN_POINT('',(181.574975961468,5.93046172357687,44.4495970221434));
#19921=CARTESIAN_POINT('Ctrl Pts',(181.549583741031,6.,44.45));
#19922=CARTESIAN_POINT('Ctrl Pts',(181.549707610205,5.99966078193585,44.45));
#19923=CARTESIAN_POINT('Ctrl Pts',(181.549833087975,5.99931715850951,44.449999977092));
#19924=CARTESIAN_POINT('Ctrl Pts',(181.549992831536,5.99887969292094,44.4499998954093));
#19925=CARTESIAN_POINT('Ctrl Pts',(181.550160009223,5.99842186860979,44.4499998099254));
#19926=CARTESIAN_POINT('Ctrl Pts',(181.550364576326,5.99786164759481,44.4499996610084));
#19927=CARTESIAN_POINT('Ctrl Pts',(181.550623975936,5.9971512589496,44.4499993237228));
#19928=CARTESIAN_POINT('Ctrl Pts',(181.550917399083,5.99634769386081,44.449998942198));
#19929=CARTESIAN_POINT('Ctrl Pts',(181.551280972928,5.99535200978955,44.4499983178149));
#19930=CARTESIAN_POINT('Ctrl Pts',(181.551715728478,5.99416138267107,44.4499971592116));
#19931=CARTESIAN_POINT('Ctrl Pts',(181.552191407404,5.9928586822711,44.4499958915495));
#19932=CARTESIAN_POINT('Ctrl Pts',(181.552751853379,5.9913238330328,44.4499939695697));
#19933=CARTESIAN_POINT('Ctrl Pts',(181.553374825605,5.9896177447235,44.4499910173912));
#19934=CARTESIAN_POINT('Ctrl Pts',(181.554306515129,5.98706619500538,44.4499866022445));
#19935=CARTESIAN_POINT('Ctrl Pts',(181.555376376442,5.98413623755719,44.4499797759452));
#19936=CARTESIAN_POINT('Ctrl Pts',(181.55647002379,5.98114113800806,44.4499703618705));
#19937=CARTESIAN_POINT('Ctrl Pts',(181.557207556768,5.97912130529461,44.4499640132147));
#19938=CARTESIAN_POINT('Ctrl Pts',(181.557954796465,5.97707488911245,44.449956536428));
#19939=CARTESIAN_POINT('Ctrl Pts',(181.558685057496,5.97507497283002,44.4499482283617));
#19940=CARTESIAN_POINT('Ctrl Pts',(181.559321396133,5.9733322754311,44.4499409888359));
#19941=CARTESIAN_POINT('Ctrl Pts',(181.559944600795,5.97162554831108,44.4499331368467));
#19942=CARTESIAN_POINT('Ctrl Pts',(181.560550795988,5.96996540673538,44.449924826463));
#19943=CARTESIAN_POINT('Ctrl Pts',(181.561117770701,5.96841267536218,44.4499170537564));
#19944=CARTESIAN_POINT('Ctrl Pts',(181.561669676874,5.96690121361503,44.4499088939209));
#19945=CARTESIAN_POINT('Ctrl Pts',(181.562219214574,5.96539624329965,44.4499002141721));
#19946=CARTESIAN_POINT('Ctrl Pts',(181.562769657243,5.96388879462565,44.4498915201296));
#19947=CARTESIAN_POINT('Ctrl Pts',(181.563320820828,5.96237937699256,44.4498822564462));
#19948=CARTESIAN_POINT('Ctrl Pts',(181.563886793199,5.96082941196163,44.4498721373903));
#19949=CARTESIAN_POINT('Ctrl Pts',(181.564499529544,5.95915137968164,44.4498611822383));
#19950=CARTESIAN_POINT('Ctrl Pts',(181.565129440981,5.95742632106529,44.4498492142267));
#19951=CARTESIAN_POINT('Ctrl Pts',(181.565773547862,5.95566239775938,44.4498361791825));
#19952=CARTESIAN_POINT('Ctrl Pts',(181.566526402788,5.95360066175229,44.4498209433614));
#19953=CARTESIAN_POINT('Ctrl Pts',(181.567298354351,5.9514866428474,44.449804231063));
#19954=CARTESIAN_POINT('Ctrl Pts',(181.568060534484,5.94939939730955,44.44978662779));
#19955=CARTESIAN_POINT('Ctrl Pts',(181.568975496117,5.9468937565782,44.4497654958833));
#19956=CARTESIAN_POINT('Ctrl Pts',(181.569874756927,5.94443113354704,44.4497430857959));
#19957=CARTESIAN_POINT('Ctrl Pts',(181.57069080425,5.94219640517704,44.4497215555745));
#19958=CARTESIAN_POINT('Ctrl Pts',(181.571319793182,5.94047393226165,44.4497049606166));
#19959=CARTESIAN_POINT('Ctrl Pts',(181.571898558316,5.93888900550459,44.4496889382245));
#19960=CARTESIAN_POINT('Ctrl Pts',(181.57240308679,5.9375073781912,44.4496745471917));
#19961=CARTESIAN_POINT('Ctrl Pts',(181.572861384492,5.93625235165496,44.4496614748328));
#19962=CARTESIAN_POINT('Ctrl Pts',(181.573258107921,5.93516594803045,44.449649769955));
#19963=CARTESIAN_POINT('Ctrl Pts',(181.573588041993,5.93426244475501,44.4496398703448));
#19964=CARTESIAN_POINT('Ctrl Pts',(181.573897632268,5.93341465165737,44.4496305811463));
#19965=CARTESIAN_POINT('Ctrl Pts',(181.574148214464,5.93272845006904,44.4496228920196));
#19966=CARTESIAN_POINT('Ctrl Pts',(181.574350823487,5.93217361966883,44.4496166195959));
#19967=CARTESIAN_POINT('Ctrl Pts',(181.574540416331,5.93165443315097,44.4496107501305));
#19968=CARTESIAN_POINT('Ctrl Pts',(181.574687916207,5.93125051528096,44.4496061233658));
#19969=CARTESIAN_POINT('Ctrl Pts',(181.574818135509,5.93089391886264,44.4496020159299));
#19970=CARTESIAN_POINT('Ctrl Pts',(181.574872642657,5.93074465486329,44.4496002966408));
#19971=CARTESIAN_POINT('Ctrl Pts',(181.574924327433,5.93060311971796,44.4495986609941));
#19972=CARTESIAN_POINT('Ctrl Pts',(181.574975961468,5.93046172357687,44.4495970221434));
#19973=CARTESIAN_POINT('',(181.949550764146,6.06724050219233,44.4278251806365));
#19974=CARTESIAN_POINT('Ctrl Pts',(181.949550764146,6.06724050219233,44.4278251806365));
#19975=CARTESIAN_POINT('Ctrl Pts',(181.824692496587,6.02164757598718,44.4350824611388));
#19976=CARTESIAN_POINT('Ctrl Pts',(181.699834229027,5.97605464978202,44.4423397416411));
#19977=CARTESIAN_POINT('Ctrl Pts',(181.574975961468,5.93046172357687,44.4495970221434));
#19978=CARTESIAN_POINT('',(181.7625,6.5830951894845,44.45));
#19979=CARTESIAN_POINT('Ctrl Pts',(181.949550764146,6.06724050219233,44.4278251806365));
#19980=CARTESIAN_POINT('Ctrl Pts',(181.94902079535,6.06873325846841,44.4279526270998));
#19981=CARTESIAN_POINT('Ctrl Pts',(181.948489242811,6.0702301556008,44.4280799229918));
#19982=CARTESIAN_POINT('Ctrl Pts',(181.947901535215,6.07188520706795,44.4282199372542));
#19983=CARTESIAN_POINT('Ctrl Pts',(181.94728649341,6.07361723477844,44.428366463563));
#19984=CARTESIAN_POINT('Ctrl Pts',(181.946609960367,6.07552244719632,44.4285269212254));
#19985=CARTESIAN_POINT('Ctrl Pts',(181.945828468642,6.07772300647724,44.4287109043704));
#19986=CARTESIAN_POINT('Ctrl Pts',(181.945018113731,6.08000484000598,44.4289016826478));
#19987=CARTESIAN_POINT('Ctrl Pts',(181.944094971134,6.08260405095877,44.4291177455792));
#19988=CARTESIAN_POINT('Ctrl Pts',(181.943030000191,6.08560145944807,44.4293644327469));
#19989=CARTESIAN_POINT('Ctrl Pts',(181.941916949163,6.08873419149441,44.4296222570636));
#19990=CARTESIAN_POINT('Ctrl Pts',(181.940649054564,6.09230165446145,44.4299135097798));
#19991=CARTESIAN_POINT('Ctrl Pts',(181.939212886804,6.09633987852072,44.4302387811672));
#19992=CARTESIAN_POINT('Ctrl Pts',(181.937693398372,6.10061238408365,44.4305829234911));
#19993=CARTESIAN_POINT('Ctrl Pts',(181.93598564529,6.10541155385979,44.4309650964571));
#19994=CARTESIAN_POINT('Ctrl Pts',(181.934093970544,6.11072251487221,44.4313805150329));
#19995=CARTESIAN_POINT('Ctrl Pts',(181.932049062151,6.11646368616331,44.4318295842683));
#19996=CARTESIAN_POINT('Ctrl Pts',(181.929789367954,6.12280248007158,44.4323174065243));
#19997=CARTESIAN_POINT('Ctrl Pts',(181.927341610279,6.12966028043394,44.4328328324238));
#19998=CARTESIAN_POINT('Ctrl Pts',(181.924565122129,6.13743907390991,44.4334174793095));
#19999=CARTESIAN_POINT('Ctrl Pts',(181.921546914366,6.1458848393179,44.4340374388843));
#20000=CARTESIAN_POINT('Ctrl Pts',(181.918349533181,6.15481772771552,44.4346724941065));
#20001=CARTESIAN_POINT('Ctrl Pts',(181.913396618503,6.16865525020576,44.4356562286534));
#20002=CARTESIAN_POINT('Ctrl Pts',(181.908015230853,6.18365673017568,44.4366745490118));
#20003=CARTESIAN_POINT('Ctrl Pts',(181.902486840944,6.19902659072339,44.4376570855153));
#20004=CARTESIAN_POINT('Ctrl Pts',(181.898955195236,6.2088451641123,44.4382847494253));
#20005=CARTESIAN_POINT('Ctrl Pts',(181.895364682588,6.21881124267631,44.4388980670532));
#20006=CARTESIAN_POINT('Ctrl Pts',(181.891781419326,6.22874060155642,44.4394848412838));
#20007=CARTESIAN_POINT('Ctrl Pts',(181.888422110018,6.23804937550653,44.440034942125));
#20008=CARTESIAN_POINT('Ctrl Pts',(181.885069687638,6.24732450257578,44.4405617369166));
#20009=CARTESIAN_POINT('Ctrl Pts',(181.881762187736,6.25646133484379,44.4410603836474));
#20010=CARTESIAN_POINT('Ctrl Pts',(181.878871956411,6.26444547985546,44.4414961219527));
#20011=CARTESIAN_POINT('Ctrl Pts',(181.876016047721,6.27232401048766,44.4419104549414));
#20012=CARTESIAN_POINT('Ctrl Pts',(181.873204044664,6.2800714641089,44.4423033601437));
#20013=CARTESIAN_POINT('Ctrl Pts',(181.870561055752,6.28735326060817,44.4426726499603));
#20014=CARTESIAN_POINT('Ctrl Pts',(181.867956945665,6.29451902766672,44.4430230545958));
#20015=CARTESIAN_POINT('Ctrl Pts',(181.865383784351,6.30159180112175,44.4433567463113));
#20016=CARTESIAN_POINT('Ctrl Pts',(181.862914409609,6.30837929945407,44.4436769788165));
#20017=CARTESIAN_POINT('Ctrl Pts',(181.860473628296,6.31508091628731,44.4439818551709));
#20018=CARTESIAN_POINT('Ctrl Pts',(181.858037986204,6.32176249133492,44.4442748222071));
#20019=CARTESIAN_POINT('Ctrl Pts',(181.855552642216,6.32858041110422,44.4445737675507));
#20020=CARTESIAN_POINT('Ctrl Pts',(181.85306986129,6.33538518338409,44.4448606695743));
#20021=CARTESIAN_POINT('Ctrl Pts',(181.85055859404,6.34226352247208,44.4451387828648));
#20022=CARTESIAN_POINT('Ctrl Pts',(181.847967136051,6.34936150329404,44.4454257769744));
#20023=CARTESIAN_POINT('Ctrl Pts',(181.845345405643,6.35653763295404,44.4457033474357));
#20024=CARTESIAN_POINT('Ctrl Pts',(181.84267965057,6.36383078704426,44.4459718736454));
#20025=CARTESIAN_POINT('Ctrl Pts',(181.839865757128,6.37152922816241,44.4462553220942));
#20026=CARTESIAN_POINT('Ctrl Pts',(181.837002917605,6.37935774694832,44.4465286150796));
#20027=CARTESIAN_POINT('Ctrl Pts',(181.834095833498,6.38730452968734,44.4467898321551));
#20028=CARTESIAN_POINT('Ctrl Pts',(181.830966994874,6.39585749886745,44.4470709750614));
#20029=CARTESIAN_POINT('Ctrl Pts',(181.827787062508,6.40454701082733,44.4473380241507));
#20030=CARTESIAN_POINT('Ctrl Pts',(181.824583454508,6.41329920717486,44.4475873899933));
#20031=CARTESIAN_POINT('Ctrl Pts',(181.820974942929,6.42315759242375,44.4478682731508));
#20032=CARTESIAN_POINT('Ctrl Pts',(181.817336668825,6.43309474070496,44.4481265525157));
#20033=CARTESIAN_POINT('Ctrl Pts',(181.8137310421,6.44294165689817,44.4483579274519));
#20034=CARTESIAN_POINT('Ctrl Pts',(181.806940176017,6.46148741725839,44.4487937008491));
#20035=CARTESIAN_POINT('Ctrl Pts',(181.800267516052,6.47970668562816,44.4491309639821));
#20036=CARTESIAN_POINT('Ctrl Pts',(181.794215639515,6.49623650830588,44.449371076666));
#20037=CARTESIAN_POINT('Ctrl Pts',(181.791120505867,6.50469041678578,44.4494938783859));
#20038=CARTESIAN_POINT('Ctrl Pts',(181.788188347131,6.51270076759385,44.4495920666799));
#20039=CARTESIAN_POINT('Ctrl Pts',(181.785475746618,6.52011386975146,44.4496700038562));
#20040=CARTESIAN_POINT('Ctrl Pts',(181.783031242769,6.5267943067218,44.4497402382038));
#20041=CARTESIAN_POINT('Ctrl Pts',(181.780765274131,6.53298908189307,44.4497941150971));
#20042=CARTESIAN_POINT('Ctrl Pts',(181.778704924533,6.53862447797697,44.449835858424));
#20043=CARTESIAN_POINT('Ctrl Pts',(181.77677798253,6.54389498228005,44.4498748988714));
#20044=CARTESIAN_POINT('Ctrl Pts',(181.775031043383,6.54867578880741,44.4499033746775));
#20045=CARTESIAN_POINT('Ctrl Pts',(181.773470463133,6.55294946200246,44.4499247770501));
#20046=CARTESIAN_POINT('Ctrl Pts',(181.772018885453,6.55692462997286,44.4499446845213));
#20047=CARTESIAN_POINT('Ctrl Pts',(181.770728582699,6.56046091928445,44.4499584916947));
#20048=CARTESIAN_POINT('Ctrl Pts',(181.769589326039,6.56358602529954,44.4499685877935));
#20049=CARTESIAN_POINT('Ctrl Pts',(181.768484615927,6.56661636634274,44.4499783777406));
#20050=CARTESIAN_POINT('Ctrl Pts',(181.767522032915,6.56925979952929,44.4499846840721));
#20051=CARTESIAN_POINT('Ctrl Pts',(181.766676133959,6.57158547767921,44.4499890998665));
#20052=CARTESIAN_POINT('Ctrl Pts',(181.765852458422,6.57385005571547,44.4499933996493));
#20053=CARTESIAN_POINT('Ctrl Pts',(181.765139502996,6.5758131168861,44.4499959037341));
#20054=CARTESIAN_POINT('Ctrl Pts',(181.764496879593,6.57758458469779,44.4499975077911));
#20055=CARTESIAN_POINT('Ctrl Pts',(181.763874348493,6.57930066568948,44.4499990616955));
#20056=CARTESIAN_POINT('Ctrl Pts',(181.763317868564,6.5808368131827,44.4499997670013));
#20057=CARTESIAN_POINT('Ctrl Pts',(181.762773707633,6.58233938708511,44.4499999531776));
#20058=CARTESIAN_POINT('Ctrl Pts',(181.762682266775,6.58259187975397,44.4499999844627));
#20059=CARTESIAN_POINT('Ctrl Pts',(181.762591132757,6.58284353633941,44.45));
#20060=CARTESIAN_POINT('Ctrl Pts',(181.7625,6.5830951894845,44.45));
#20061=CARTESIAN_POINT('',(181.656041870516,6.29154759474225,44.45));
#20062=CARTESIAN_POINT('Ctrl Pts',(181.949550764146,6.06724050219231,44.4278251806365));
#20063=CARTESIAN_POINT('Ctrl Pts',(182.122029380922,5.58142220595409,44.3863476637473));
#20064=CARTESIAN_POINT('Ctrl Pts',(182.295726981729,5.05523944602546,44.2805738182329));
#20065=CARTESIAN_POINT('Ctrl Pts',(182.504123999729,4.15716068129026,43.9875888528751));
#20066=CARTESIAN_POINT('Ctrl Pts',(182.562500000088,3.77824139277389,43.8274217463149));
#20067=CARTESIAN_POINT('Ctrl Pts',(182.5625,3.42868316199153,43.6499999996042));
#20068=CARTESIAN_POINT('Ctrl Pts',(181.824692496587,6.02164757598716,44.4350824611388));
#20069=CARTESIAN_POINT('Ctrl Pts',(181.998734032867,5.53583221576672,44.4055514751814));
#20070=CARTESIAN_POINT('Ctrl Pts',(182.178886012691,5.01057273132897,44.3122210149538));
#20071=CARTESIAN_POINT('Ctrl Pts',(182.407104469443,4.11610731539274,44.0359022508337));
#20072=CARTESIAN_POINT('Ctrl Pts',(182.476676711275,3.73937765462172,43.8811967422844));
#20073=CARTESIAN_POINT('Ctrl Pts',(182.489526917701,3.39266652940122,43.7061729265265));
#20074=CARTESIAN_POINT('Ctrl Pts',(181.699834229027,5.97605464978202,44.4423397416411));
#20075=CARTESIAN_POINT('Ctrl Pts',(181.875666121718,5.49026860678201,44.424762745888));
#20076=CARTESIAN_POINT('Ctrl Pts',(182.062102046114,4.96591082303663,44.3438616250727));
#20077=CARTESIAN_POINT('Ctrl Pts',(182.310082295719,4.07505300028109,44.0842157500705));
#20078=CARTESIAN_POINT('Ctrl Pts',(182.390946147939,3.70051482158828,43.934941903938));
#20079=CARTESIAN_POINT('Ctrl Pts',(182.416553835402,3.3566498968109,43.7623458534489));
#20080=CARTESIAN_POINT('Ctrl Pts',(181.574975961468,5.93046172357687,44.4495970221434));
#20081=CARTESIAN_POINT('Ctrl Pts',(181.752370773663,5.44467861659464,44.4439665573221));
#20082=CARTESIAN_POINT('Ctrl Pts',(181.945261077076,4.92124410834014,44.3755088217936));
#20083=CARTESIAN_POINT('Ctrl Pts',(182.213062765432,4.03399963438357,44.1325291480292));
#20084=CARTESIAN_POINT('Ctrl Pts',(182.305122859126,3.66165108343612,43.9887168999075));
#20085=CARTESIAN_POINT('Ctrl Pts',(182.343580753104,3.32063326422058,43.8185187803712));
#20086=CARTESIAN_POINT('',(182.343580753104,3.3206332642207,43.8185187803713));
#20087=CARTESIAN_POINT('Ctrl Pts',(181.574975961468,5.93046172357687,44.4495970221434));
#20088=CARTESIAN_POINT('Ctrl Pts',(181.752370773663,5.44467861659464,44.4439665573221));
#20089=CARTESIAN_POINT('Ctrl Pts',(181.945261077076,4.92124410834014,44.3755088217936));
#20090=CARTESIAN_POINT('Ctrl Pts',(182.213062765432,4.03399963438357,44.1325291480292));
#20091=CARTESIAN_POINT('Ctrl Pts',(182.305122859126,3.66165108343612,43.9887168999075));
#20092=CARTESIAN_POINT('Ctrl Pts',(182.343580753104,3.32063326422058,43.8185187803712));
#20093=CARTESIAN_POINT('',(182.5625,3.42868316190269,43.6499999997796));
#20094=CARTESIAN_POINT('',(182.343580753104,3.3206332642207,43.8185187803713));
#20095=CARTESIAN_POINT('Ctrl Pts',(182.5625,3.42868316199153,43.6499999996042));
#20096=CARTESIAN_POINT('Ctrl Pts',(182.562500000088,3.77824139277389,43.8274217463149));
#20097=CARTESIAN_POINT('Ctrl Pts',(182.504123999729,4.15716068129026,43.9875888528751));
#20098=CARTESIAN_POINT('Ctrl Pts',(182.295726981729,5.05523944602546,44.2805738182329));
#20099=CARTESIAN_POINT('Ctrl Pts',(182.122029380922,5.58142220595409,44.3863476637473));
#20100=CARTESIAN_POINT('Ctrl Pts',(181.949550764146,6.06724050219231,44.4278251806365));
#20101=CARTESIAN_POINT('Origin',(182.4625,6.00000000000001,38.45));
#20102=CARTESIAN_POINT('',(182.3625,0.800000000000003,41.4433259094192));
#20103=CARTESIAN_POINT('',(182.5625,0.973333333333333,41.3435483791052));
#20104=CARTESIAN_POINT('',(182.3625,0.800000000000003,41.4433259094192));
#20105=CARTESIAN_POINT('',(182.5625,3.10645162089482,43.4766666666667));
#20106=CARTESIAN_POINT('Origin',(182.5625,6.00000000000001,38.45));
#20107=CARTESIAN_POINT('',(182.3625,3.00667409058085,43.65));
#20108=CARTESIAN_POINT('',(182.5625,3.10645162089482,43.4766666666667));
#20109=CARTESIAN_POINT('Origin',(182.3625,6.00000000000001,38.45));
#20110=CARTESIAN_POINT('Ctrl Pts',(182.5625,3.42868316199165,43.6499999996043));
#20111=CARTESIAN_POINT('Ctrl Pts',(182.5625,3.31801931336449,43.593831465749));
#20112=CARTESIAN_POINT('Ctrl Pts',(182.5625,3.21069598181731,43.5366738486782));
#20113=CARTESIAN_POINT('Ctrl Pts',(182.5625,3.10645162089483,43.4766666666667));
#20114=CARTESIAN_POINT('Ctrl Pts',(182.489526917701,3.39266652940134,43.7061729265266));
#20115=CARTESIAN_POINT('Ctrl Pts',(182.493585276875,3.28290392767115,43.650766682816));
#20116=CARTESIAN_POINT('Ctrl Pts',(182.495833333333,3.17639835547358,43.5938538537616));
#20117=CARTESIAN_POINT('Ctrl Pts',(182.495833333333,3.07319244412351,43.5344444444445));
#20118=CARTESIAN_POINT('Ctrl Pts',(182.416553835402,3.35664989681102,43.762345853449));
#20119=CARTESIAN_POINT('Ctrl Pts',(182.424670553749,3.24778854197781,43.7077018998829));
#20120=CARTESIAN_POINT('Ctrl Pts',(182.429166666667,3.14210072912985,43.6510338588451));
#20121=CARTESIAN_POINT('Ctrl Pts',(182.429166666667,3.03993326735218,43.5922222222222));
#20122=CARTESIAN_POINT('Ctrl Pts',(182.343580753104,3.32063326422071,43.8185187803713));
#20123=CARTESIAN_POINT('Ctrl Pts',(182.355755830624,3.21267315628446,43.7646371169499));
#20124=CARTESIAN_POINT('Ctrl Pts',(182.3625,3.10780310278612,43.7082138639285));
#20125=CARTESIAN_POINT('Ctrl Pts',(182.3625,3.00667409058086,43.65));
#20126=CARTESIAN_POINT('Ctrl Pts',(182.5625,3.10645162089483,43.4766666666667));
#20127=CARTESIAN_POINT('Ctrl Pts',(182.5625,3.21069598181731,43.5366738486782));
#20128=CARTESIAN_POINT('Ctrl Pts',(182.5625,3.31801931336449,43.593831465749));
#20129=CARTESIAN_POINT('Ctrl Pts',(182.5625,3.42868316199165,43.6499999996043));
#20130=CARTESIAN_POINT('Ctrl Pts',(182.343580753104,3.32063326422071,43.8185187803713));
#20131=CARTESIAN_POINT('Ctrl Pts',(182.355755830624,3.21267315628446,43.7646371169499));
#20132=CARTESIAN_POINT('Ctrl Pts',(182.3625,3.10780310278612,43.7082138639285));
#20133=CARTESIAN_POINT('Ctrl Pts',(182.3625,3.00667409058086,43.65));
#20134=CARTESIAN_POINT('Ctrl Pts',(182.5625,0.800000001098831,41.0213168393936));
#20135=CARTESIAN_POINT('Ctrl Pts',(182.562500000222,0.638342237723523,40.7028169780214));
#20136=CARTESIAN_POINT('Ctrl Pts',(182.510237346477,0.488965591972109,40.349303524625));
#20137=CARTESIAN_POINT('Ctrl Pts',(182.334919667211,0.201305187631971,39.5253711428458));
#20138=CARTESIAN_POINT('Ctrl Pts',(182.135056358579,0.0667849130182742,
38.9052706332517));
#20139=CARTESIAN_POINT('Ctrl Pts',(181.949550208499,0.0221746857420428,
38.3827579327069));
#20140=CARTESIAN_POINT('Ctrl Pts',(182.489526917752,0.743827074166946,41.0573334719727));
#20141=CARTESIAN_POINT('Ctrl Pts',(182.477698497965,0.584280425725848,40.7414573298172));
#20142=CARTESIAN_POINT('Ctrl Pts',(182.415138024714,0.439988962986447,40.3899691894989));
#20143=CARTESIAN_POINT('Ctrl Pts',(182.220050603944,0.166732430848469,39.5697265255869));
#20144=CARTESIAN_POINT('Ctrl Pts',(182.011622935248,0.0465939131825897,
38.9509143970108));
#20145=CARTESIAN_POINT('Ctrl Pts',(181.824691935409,0.0149174437260072,
38.4283508582629));
#20146=CARTESIAN_POINT('Ctrl Pts',(182.416553835504,0.68765414723506,41.0933501045517));
#20147=CARTESIAN_POINT('Ctrl Pts',(182.393341358808,0.53046707431298,40.7800081170217));
#20148=CARTESIAN_POINT('Ctrl Pts',(182.319938208693,0.390945991654019,40.4306566666258));
#20149=CARTESIAN_POINT('Ctrl Pts',(182.105417882415,0.132285334982405,39.6140336660972));
#20150=CARTESIAN_POINT('Ctrl Pts',(181.889203292348,0.0266495899212865,
38.9963701019499));
#20151=CARTESIAN_POINT('Ctrl Pts',(181.69983366232,0.00766020170997153,
38.4739437838189));
#20152=CARTESIAN_POINT('Ctrl Pts',(182.343580753256,0.631481220303175,41.1293667371307));
#20153=CARTESIAN_POINT('Ctrl Pts',(182.308539856551,0.476405262315305,40.8186484688175));
#20154=CARTESIAN_POINT('Ctrl Pts',(182.22483888693,0.341969362668358,40.4713223314997));
#20155=CARTESIAN_POINT('Ctrl Pts',(181.990548819148,0.0977125781989031,
39.6583890488383));
#20156=CARTESIAN_POINT('Ctrl Pts',(181.765769869017,0.00645859008560202,
39.042013865709));
#20157=CARTESIAN_POINT('Ctrl Pts',(181.57497538923,0.000402959693935889,
38.5195367093749));
#20158=CARTESIAN_POINT('',(182.5625,0.800000000612018,41.0213168396403));
#20159=CARTESIAN_POINT('Ctrl Pts',(181.949550208499,0.0221746857420428,
38.3827579327069));
#20160=CARTESIAN_POINT('Ctrl Pts',(182.135056358579,0.0667849130182742,
38.9052706332517));
#20161=CARTESIAN_POINT('Ctrl Pts',(182.334919667211,0.201305187631971,39.5253711428458));
#20162=CARTESIAN_POINT('Ctrl Pts',(182.510237346477,0.488965591972109,40.349303524625));
#20163=CARTESIAN_POINT('Ctrl Pts',(182.562500000222,0.638342237723523,40.7028169780214));
#20164=CARTESIAN_POINT('Ctrl Pts',(182.5625,0.800000001098831,41.0213168393936));
#20165=CARTESIAN_POINT('',(182.343580753256,0.631481220303007,41.1293667371304));
#20166=CARTESIAN_POINT('',(182.5625,0.800000000612018,41.0213168396403));
#20167=CARTESIAN_POINT('Ctrl Pts',(182.343580753256,0.631481220303175,41.1293667371307));
#20168=CARTESIAN_POINT('Ctrl Pts',(182.308539856551,0.476405262315305,40.8186484688175));
#20169=CARTESIAN_POINT('Ctrl Pts',(182.22483888693,0.341969362668358,40.4713223314997));
#20170=CARTESIAN_POINT('Ctrl Pts',(181.990548819148,0.0977125781989031,
39.6583890488383));
#20171=CARTESIAN_POINT('Ctrl Pts',(181.765769869017,0.00645859008560202,
39.042013865709));
#20172=CARTESIAN_POINT('Ctrl Pts',(181.57497538923,0.000402959693935889,
38.5195367093749));
#20173=CARTESIAN_POINT('Ctrl Pts',(182.5625,0.973333333333336,41.3435483791052));
#20174=CARTESIAN_POINT('Ctrl Pts',(182.5625,0.914909659101875,41.242054884846));
#20175=CARTESIAN_POINT('Ctrl Pts',(182.5625,0.857236572714185,41.1340849474454));
#20176=CARTESIAN_POINT('Ctrl Pts',(182.5625,0.800000001098665,41.0213168393933));
#20177=CARTESIAN_POINT('Ctrl Pts',(182.495833333333,0.915555555555558,41.3768075558765));
#20178=CARTESIAN_POINT('Ctrl Pts',(182.495833333333,0.857713879611461,41.2763251079203));
#20179=CARTESIAN_POINT('Ctrl Pts',(182.49366244611,0.800286860789319,41.169183196029));
#20180=CARTESIAN_POINT('Ctrl Pts',(182.489526917752,0.743827074166782,41.0573334719723));
#20181=CARTESIAN_POINT('Ctrl Pts',(182.429166666667,0.857777777777781,41.4100667326478));
#20182=CARTESIAN_POINT('Ctrl Pts',(182.429166666667,0.800518100121046,41.3105953309945));
#20183=CARTESIAN_POINT('Ctrl Pts',(182.42482489222,0.743337148864453,41.2042814446125));
#20184=CARTESIAN_POINT('Ctrl Pts',(182.416553835504,0.687654147234898,41.0933501045513));
#20185=CARTESIAN_POINT('Ctrl Pts',(182.3625,0.800000000000004,41.4433259094192));
#20186=CARTESIAN_POINT('Ctrl Pts',(182.3625,0.743322320630632,41.3448655540688));
#20187=CARTESIAN_POINT('Ctrl Pts',(182.355987338329,0.686387436939587,41.239379693196));
#20188=CARTESIAN_POINT('Ctrl Pts',(182.343580753256,0.631481220303014,41.1293667371304));
#20189=CARTESIAN_POINT('Ctrl Pts',(182.5625,0.800000001098665,41.0213168393933));
#20190=CARTESIAN_POINT('Ctrl Pts',(182.5625,0.857236572714185,41.1340849474454));
#20191=CARTESIAN_POINT('Ctrl Pts',(182.5625,0.914909659101875,41.242054884846));
#20192=CARTESIAN_POINT('Ctrl Pts',(182.5625,0.973333333333336,41.3435483791052));
#20193=CARTESIAN_POINT('Ctrl Pts',(182.3625,0.800000000000004,41.4433259094192));
#20194=CARTESIAN_POINT('Ctrl Pts',(182.3625,0.743322320630632,41.3448655540688));
#20195=CARTESIAN_POINT('Ctrl Pts',(182.355987338329,0.686387436939587,41.239379693196));
#20196=CARTESIAN_POINT('Ctrl Pts',(182.343580753256,0.631481220303014,41.1293667371304));
#20197=CARTESIAN_POINT('Origin',(181.7625,0.800000000000001,3.35000000000001));
#20198=CARTESIAN_POINT('',(181.949550200389,0.0221746837918946,-101.88275790988));
#20199=CARTESIAN_POINT('Ctrl Pts',(181.949550200389,0.0221746837918912,
-101.88275790988));
#20200=CARTESIAN_POINT('Ctrl Pts',(181.949020231057,0.0220472376058877,
-101.881265152351));
#20201=CARTESIAN_POINT('Ctrl Pts',(181.948488677977,0.0219199419923545,
-101.879768253967));
#20202=CARTESIAN_POINT('Ctrl Pts',(181.947900969848,0.0217799280541142,
-101.878113201481));
#20203=CARTESIAN_POINT('Ctrl Pts',(181.947285927459,0.0216334020783753,
-101.876381172632));
#20204=CARTESIAN_POINT('Ctrl Pts',(181.946609393835,0.0214729447980497,
-101.874475959315));
#20205=CARTESIAN_POINT('Ctrl Pts',(181.945827901584,0.0212889621299003,
-101.872275399603));
#20206=CARTESIAN_POINT('Ctrl Pts',(181.945017546083,0.0210981843364628,
-101.869993565502));
#20207=CARTESIAN_POINT('Ctrl Pts',(181.944094402945,0.0208821219884184,
-101.867394354444));
#20208=CARTESIAN_POINT('Ctrl Pts',(181.943029431607,0.0206354355477969,
-101.864396946535));
#20209=CARTESIAN_POINT('Ctrl Pts',(181.941916380075,0.0203776119700361,
-101.861264214841));
#20210=CARTESIAN_POINT('Ctrl Pts',(181.940648485108,0.0200863601446586,
-101.857696752903));
#20211=CARTESIAN_POINT('Ctrl Pts',(181.939212317266,0.0197610898408669,
-101.853658530765));
#20212=CARTESIAN_POINT('Ctrl Pts',(181.937692828547,0.0194169486180327,
-101.849386026672));
#20213=CARTESIAN_POINT('Ctrl Pts',(181.93598507545,0.0190347769592833,-101.844586859225));
#20214=CARTESIAN_POINT('Ctrl Pts',(181.934093401175,0.0186193599318965,
-101.839275901635));
#20215=CARTESIAN_POINT('Ctrl Pts',(181.93204849278,0.0181702922577936,-101.833534732605));
#20216=CARTESIAN_POINT('Ctrl Pts',(181.929788799043,0.0176824718261296,
-101.827195941937));
#20217=CARTESIAN_POINT('Ctrl Pts',(181.927341042605,0.0171670480409611,
-101.82033814611));
#20218=CARTESIAN_POINT('Ctrl Pts',(181.924564553008,0.0165824029531123,
-101.812559349791));
#20219=CARTESIAN_POINT('Ctrl Pts',(181.921546344304,0.0159624454782107,
-101.804113581838));
#20220=CARTESIAN_POINT('Ctrl Pts',(181.91834896333,0.0153273927115106,-101.795180692153));
#20221=CARTESIAN_POINT('Ctrl Pts',(181.913396100735,0.0143436722478956,
-101.781343312265));
#20222=CARTESIAN_POINT('Ctrl Pts',(181.908014776974,0.0133253675338641,
-101.766342002379));
#20223=CARTESIAN_POINT('Ctrl Pts',(181.902486455809,0.0123428460364121,
-101.750972317255));
#20224=CARTESIAN_POINT('Ctrl Pts',(181.89895482528,0.0117151866054473,-101.741153776038));
#20225=CARTESIAN_POINT('Ctrl Pts',(181.895364328797,0.0111018734427425,
-101.731187729355));
#20226=CARTESIAN_POINT('Ctrl Pts',(181.891781082577,0.0105151035721518,
-101.721258401538));
#20227=CARTESIAN_POINT('Ctrl Pts',(181.888421789245,0.009965006818473,-101.71194965671));
#20228=CARTESIAN_POINT('Ctrl Pts',(181.885069383611,0.00943821602199506,
-101.70267455804));
#20229=CARTESIAN_POINT('Ctrl Pts',(181.881761901085,0.00893957313635096,
-101.69353775326));
#20230=CARTESIAN_POINT('Ctrl Pts',(181.878871682462,0.00850383781729341,
-101.685553625418));
#20231=CARTESIAN_POINT('Ctrl Pts',(181.876015787016,0.00808950773794182,
-101.677675111449));
#20232=CARTESIAN_POINT('Ctrl Pts',(181.873203797631,0.00769660533975813,
-101.669927674095));
#20233=CARTESIAN_POINT('Ctrl Pts',(181.870560822923,0.00732731834799652,
-101.662645896615));
#20234=CARTESIAN_POINT('Ctrl Pts',(181.867956727377,0.00697691642498478,
-101.655480148105));
#20235=CARTESIAN_POINT('Ctrl Pts',(181.865383580778,0.00664322728912792,
-101.64840739288));
#20236=CARTESIAN_POINT('Ctrl Pts',(181.862914219001,0.00632299710939984,
-101.641619908862));
#20237=CARTESIAN_POINT('Ctrl Pts',(181.86047345084,0.00601812297287069,
-101.634918306135));
#20238=CARTESIAN_POINT('Ctrl Pts',(181.858037821854,0.00572515802433116,
-101.628236745118));
#20239=CARTESIAN_POINT('Ctrl Pts',(181.855552491816,0.0054262148804763,
-101.621418841249));
#20240=CARTESIAN_POINT('Ctrl Pts',(181.853069724786,0.00513931491516174,
-101.614614084804));
#20241=CARTESIAN_POINT('Ctrl Pts',(181.850558471049,0.00486120351446528,
-101.60773576152));
#20242=CARTESIAN_POINT('Ctrl Pts',(181.847967027646,0.00457421142590764,
-101.60063779876));
#20243=CARTESIAN_POINT('Ctrl Pts',(181.845345311431,0.00429664280136511,
-101.593461687163));
#20244=CARTESIAN_POINT('Ctrl Pts',(181.842679569903,0.0040281182289359,
-101.586168551203));
#20245=CARTESIAN_POINT('Ctrl Pts',(181.839865690715,0.00374467150392575,
-101.578470129103));
#20246=CARTESIAN_POINT('Ctrl Pts',(181.83700286472,0.00347138002015111,
-101.570641629404));
#20247=CARTESIAN_POINT('Ctrl Pts',(181.834095793202,0.0032101642241178,
-101.56269486586));
#20248=CARTESIAN_POINT('Ctrl Pts',(181.830966968037,0.00292902268659486,
-101.554141917091));
#20249=CARTESIAN_POINT('Ctrl Pts',(181.827787048038,0.00266197470938195,
-101.545452425659));
#20250=CARTESIAN_POINT('Ctrl Pts',(181.824583451151,0.00241260974534963,
-101.536700249963));
#20251=CARTESIAN_POINT('Ctrl Pts',(181.820974951551,0.00213172753559789,
-101.526841886502));
#20252=CARTESIAN_POINT('Ctrl Pts',(181.817336687823,0.00187344882906896,
-101.516904760142));
#20253=CARTESIAN_POINT('Ctrl Pts',(181.813731069805,0.00164207432593222,
-101.507057866022));
#20254=CARTESIAN_POINT('Ctrl Pts',(181.806940226809,0.00120630217362233,
-101.488512165496));
#20255=CARTESIAN_POINT('Ctrl Pts',(181.800267583721,0.000869039289859969,
-101.470292956922));
#20256=CARTESIAN_POINT('Ctrl Pts',(181.794215716949,0.000628926406277541,
-101.453763189425));
#20257=CARTESIAN_POINT('Ctrl Pts',(181.791120585805,0.000506124485427283,
-101.445309302364));
#20258=CARTESIAN_POINT('Ctrl Pts',(181.788188427994,0.000407935916206988,
-101.437298972468));
#20259=CARTESIAN_POINT('Ctrl Pts',(181.785475826965,0.000329998452306857,
-101.429885890493));
#20260=CARTESIAN_POINT('Ctrl Pts',(181.783031322716,0.000259763847384077,
-101.423205471888));
#20261=CARTESIAN_POINT('Ctrl Pts',(181.780765352501,0.000205886685921585,
-101.417010714464));
#20262=CARTESIAN_POINT('Ctrl Pts',(181.778705000268,0.000164143110408577,
-101.411375335315));
#20263=CARTESIAN_POINT('Ctrl Pts',(181.776778055821,0.000125102430976801,
-101.406104846907));
#20264=CARTESIAN_POINT('Ctrl Pts',(181.775031113303,9.66264096144005E-5,
-101.401324055554));
#20265=CARTESIAN_POINT('Ctrl Pts',(181.773470528856,7.52238512622405E-5,
-101.397050396643));
#20266=CARTESIAN_POINT('Ctrl Pts',(181.772018947239,5.53162068281227E-5,
-101.393075241868));
#20267=CARTESIAN_POINT('Ctrl Pts',(181.770728639844,4.15088856209883E-5,
-101.389538965001));
#20268=CARTESIAN_POINT('Ctrl Pts',(181.769589377915,3.1412666232411E-5,
-101.386413870535));
#20269=CARTESIAN_POINT('Ctrl Pts',(181.768484662701,2.16226022730055E-5,
-101.383383540712));
#20270=CARTESIAN_POINT('Ctrl Pts',(181.767522073996,1.53161792071218E-5,
-101.380740117898));
#20271=CARTESIAN_POINT('Ctrl Pts',(181.766676168814,1.09003154893372E-5,
-101.378414449133));
#20272=CARTESIAN_POINT('Ctrl Pts',(181.765852487221,6.60046517202568E-6,
-101.376149880247));
#20273=CARTESIAN_POINT('Ctrl Pts',(181.765139525231,4.09633361300762E-6,
-101.374186827287));
#20274=CARTESIAN_POINT('Ctrl Pts',(181.764496894799,2.49224690684891E-6,
-101.372415366613));
#20275=CARTESIAN_POINT('Ctrl Pts',(181.763874356865,9.38313611751158E-7,
-101.370699292469));
#20276=CARTESIAN_POINT('Ctrl Pts',(181.76331786967,2.32994581050169E-7,
-101.369163150831));
#20277=CARTESIAN_POINT('Ctrl Pts',(181.762773701049,4.68201671877111E-8,
-101.36766058165));
#20278=CARTESIAN_POINT('Ctrl Pts',(181.76268226241,1.55366010411297E-8,
-101.367408099467));
#20279=CARTESIAN_POINT('Ctrl Pts',(181.762591130575,6.66121167867262E-16,
-101.367156453271));
#20280=CARTESIAN_POINT('Ctrl Pts',(181.7625,6.66133814775094E-16,-101.366904810515));
#20281=CARTESIAN_POINT('',(182.5625,0.800000000612023,-104.52131683964));
#20282=CARTESIAN_POINT('Ctrl Pts',(182.5625,0.800000001098851,-104.521316839394));
#20283=CARTESIAN_POINT('Ctrl Pts',(182.562500000222,0.638342237723529,-104.202816978021));
#20284=CARTESIAN_POINT('Ctrl Pts',(182.51023714977,0.488966122920897,-103.849303636982));
#20285=CARTESIAN_POINT('Ctrl Pts',(182.334918859392,0.201307103612158,-103.02537106626));
#20286=CARTESIAN_POINT('Ctrl Pts',(182.135056739364,0.0667850025429474,
-102.405271696106));
#20287=CARTESIAN_POINT('Ctrl Pts',(181.949550200389,0.022174683791894,-101.88275790988));
#20288=CARTESIAN_POINT('',(182.5625,0.800000000000001,3.35000000000001));
#20289=CARTESIAN_POINT('Origin',(177.8,6.00000000000001,38.45));
#20290=CARTESIAN_POINT('',(177.8,6.,44.45));
#20291=CARTESIAN_POINT('Ctrl Pts',(181.949550265183,6.06724190764558,-107.927825300627));
#20292=CARTESIAN_POINT('Ctrl Pts',(181.9393114125,6.09608154848852,-107.930287524609));
#20293=CARTESIAN_POINT('Ctrl Pts',(181.847546692115,6.35252593990272,-107.950381345263));
#20294=CARTESIAN_POINT('Ctrl Pts',(181.770347680097,6.56142467898131,-107.95));
#20295=CARTESIAN_POINT('Ctrl Pts',(181.7625,6.58309518948447,-107.95));
#20296=CARTESIAN_POINT('Ctrl Pts',(181.824691992404,6.02164898271766,-107.935082546577));
#20297=CARTESIAN_POINT('Ctrl Pts',(181.817345081843,6.04220422326554,-107.936123736651));
#20298=CARTESIAN_POINT('Ctrl Pts',(181.752634028788,6.22404472257607,-107.952425867466));
#20299=CARTESIAN_POINT('Ctrl Pts',(181.697114000682,6.37331286135213,-107.95));
#20300=CARTESIAN_POINT('Ctrl Pts',(181.691527913677,6.38873012632298,-107.95));
#20301=CARTESIAN_POINT('Ctrl Pts',(181.699833719625,5.97605605778975,-107.942339792527));
#20302=CARTESIAN_POINT('Ctrl Pts',(181.695442063896,5.98825113903972,-107.94257327241));
#20303=CARTESIAN_POINT('Ctrl Pts',(181.655779679084,6.09746188028193,-107.947668893388));
#20304=CARTESIAN_POINT('Ctrl Pts',(181.623880321266,6.18520104372295,-107.95));
#20305=CARTESIAN_POINT('Ctrl Pts',(181.620555827354,6.19436506316149,-107.95));
#20306=CARTESIAN_POINT('Ctrl Pts',(181.574975446846,5.93046313286183,-107.949597038478));
#20307=CARTESIAN_POINT('Ctrl Pts',(181.573558332847,5.93434379914083,-107.949642016394));
#20308=CARTESIAN_POINT('Ctrl Pts',(181.56092895885,5.9689290898352,-107.950008001077));
#20309=CARTESIAN_POINT('Ctrl Pts',(181.55064664185,5.99708922609377,-107.95));
#20310=CARTESIAN_POINT('Ctrl Pts',(181.549583741031,6.,-107.95));
#20311=CARTESIAN_POINT('',(181.7625,6.58309518948447,-107.95));
#20312=CARTESIAN_POINT('',(181.949550265183,6.06724190764558,-107.927825300627));
#20313=CARTESIAN_POINT('Ctrl Pts',(181.7625,6.58309518948447,-107.95));
#20314=CARTESIAN_POINT('Ctrl Pts',(181.763041473032,6.58159997091306,-107.95));
#20315=CARTESIAN_POINT('Ctrl Pts',(181.763584461698,6.58010061545635,-107.949999490713));
#20316=CARTESIAN_POINT('Ctrl Pts',(181.764185458177,6.57844322897763,-107.949998224517));
#20317=CARTESIAN_POINT('Ctrl Pts',(181.764814399128,6.5767087791675,-107.949996899447));
#20318=CARTESIAN_POINT('Ctrl Pts',(181.765506859744,6.57480128397547,-107.949994750064));
#20319=CARTESIAN_POINT('Ctrl Pts',(181.76630768495,6.57259867099715,-107.949990938408));
#20320=CARTESIAN_POINT('Ctrl Pts',(181.76713807453,6.57031474330569,-107.949986986036));
#20321=CARTESIAN_POINT('Ctrl Pts',(181.768084909396,6.5677136941309,-107.949981251966));
#20322=CARTESIAN_POINT('Ctrl Pts',(181.769177899328,6.56471475376686,-107.949972128052));
#20323=CARTESIAN_POINT('Ctrl Pts',(181.770320208327,6.56158049199346,-107.949962592439));
#20324=CARTESIAN_POINT('Ctrl Pts',(181.771622076268,6.55801185344115,-107.949949350216));
#20325=CARTESIAN_POINT('Ctrl Pts',(181.773096798008,6.55397281294379,-107.949929814341));
#20326=CARTESIAN_POINT('Ctrl Pts',(181.774657020027,6.5496996000754,-107.949909145831));
#20327=CARTESIAN_POINT('Ctrl Pts',(181.776410610864,6.54490016320143,-107.94988140751));
#20328=CARTESIAN_POINT('Ctrl Pts',(181.778352180765,6.53958932246262,-107.949842927308));
#20329=CARTESIAN_POINT('Ctrl Pts',(181.780450879358,6.53384868238663,-107.949801332955));
#20330=CARTESIAN_POINT('Ctrl Pts',(181.782769055297,6.527510955219,-107.949747125478));
#20331=CARTESIAN_POINT('Ctrl Pts',(181.785277881027,6.5206546138659,-107.949675664339));
#20332=CARTESIAN_POINT('Ctrl Pts',(181.788122809382,6.51287974146625,-107.949594629686));
#20333=CARTESIAN_POINT('Ctrl Pts',(181.791212601148,6.50443878957439,-107.94949126786));
#20334=CARTESIAN_POINT('Ctrl Pts',(181.794481201446,6.49551117516263,-107.949360496118));
#20335=CARTESIAN_POINT('Ctrl Pts',(181.799555618821,6.48165128482589,-107.949157476373));
#20336=CARTESIAN_POINT('Ctrl Pts',(181.805059202589,6.46662336130415,-107.948887112081));
#20337=CARTESIAN_POINT('Ctrl Pts',(181.810697267405,6.45122664552554,-107.948546819801));
#20338=CARTESIAN_POINT('Ctrl Pts',(181.814293413217,6.44140610660598,-107.948329770034));
#20339=CARTESIAN_POINT('Ctrl Pts',(181.817943220182,6.43143836252728,-107.948084794035));
#20340=CARTESIAN_POINT('Ctrl Pts',(181.821578692671,6.42150762201582,-107.947815585253));
#20341=CARTESIAN_POINT('Ctrl Pts',(181.824986948131,6.41219755278633,-107.94756320202));
#20342=CARTESIAN_POINT('Ctrl Pts',(181.82838210504,6.40292137962293,-107.947289665233));
#20343=CARTESIAN_POINT('Ctrl Pts',(181.831725415348,6.3937837295531,-107.946999273444));
#20344=CARTESIAN_POINT('Ctrl Pts',(181.834646442654,6.38580022730003,-107.946745560128));
#20345=CARTESIAN_POINT('Ctrl Pts',(181.837527894586,6.37792247617696,-107.946479072676));
#20346=CARTESIAN_POINT('Ctrl Pts',(181.840360114445,6.37017591351464,-107.946202111639));
#20347=CARTESIAN_POINT('Ctrl Pts',(181.843021663982,6.36289616078084,-107.945941840348));
#20348=CARTESIAN_POINT('Ctrl Pts',(181.845639656412,6.35573249576307,-107.945672384872));
#20349=CARTESIAN_POINT('Ctrl Pts',(181.848222107743,6.34866190828394,-107.94539406601));
#20350=CARTESIAN_POINT('Ctrl Pts',(181.850700927839,6.34187505653352,-107.945126915811));
#20351=CARTESIAN_POINT('Ctrl Pts',(181.853146920829,6.33517420157077,-107.944851655773));
#20352=CARTESIAN_POINT('Ctrl Pts',(181.855583610037,6.32849354473312,-107.94456619708));
#20353=CARTESIAN_POINT('Ctrl Pts',(181.858070930426,6.32167407267557,-107.944274806933));
#20354=CARTESIAN_POINT('Ctrl Pts',(181.860551349524,6.31486792632985,-107.943972484574));
#20355=CARTESIAN_POINT('Ctrl Pts',(181.863055887233,6.30798832458689,-107.943655160345));
#20356=CARTESIAN_POINT('Ctrl Pts',(181.865640271041,6.30088939719322,-107.943327719638));
#20357=CARTESIAN_POINT('Ctrl Pts',(181.868250261284,6.29371244740061,-107.942984257084));
#20358=CARTESIAN_POINT('Ctrl Pts',(181.870899501794,6.28641857841591,-107.942621945199));
#20359=CARTESIAN_POINT('Ctrl Pts',(181.873695966718,6.27871937228751,-107.942239498805));
#20360=CARTESIAN_POINT('Ctrl Pts',(181.876536043829,6.27089020577594,-107.94183599956));
#20361=CARTESIAN_POINT('Ctrl Pts',(181.87941503676,6.26294290518415,-107.941410686167));
#20362=CARTESIAN_POINT('Ctrl Pts',(181.882513653988,6.25438934388254,-107.940952927694));
#20363=CARTESIAN_POINT('Ctrl Pts',(181.885657174003,6.24569938970116,-107.940469835403));
#20364=CARTESIAN_POINT('Ctrl Pts',(181.888818603077,6.2369469526327,-107.939964309647));
#20365=CARTESIAN_POINT('Ctrl Pts',(181.892379743607,6.22708791178712,-107.939394868355));
#20366=CARTESIAN_POINT('Ctrl Pts',(181.895963303727,6.21715035833682,-107.938796864838));
#20367=CARTESIAN_POINT('Ctrl Pts',(181.89950839463,6.20730341159208,-107.93818062638));
#20368=CARTESIAN_POINT('Ctrl Pts',(181.906183290512,6.18876302826307,-107.937020338067));
#20369=CARTESIAN_POINT('Ctrl Pts',(181.912718828949,6.17055030095437,-107.935793011526));
#20370=CARTESIAN_POINT('Ctrl Pts',(181.918632275053,6.15402777629446,-107.934616283725));
#20371=CARTESIAN_POINT('Ctrl Pts',(181.921657588146,6.14557486925797,-107.934014270963));
#20372=CARTESIAN_POINT('Ctrl Pts',(181.924519669777,6.13756600214987,-107.933426406399));
#20373=CARTESIAN_POINT('Ctrl Pts',(181.927165050345,6.13015493599256,-107.93286998997));
#20374=CARTESIAN_POINT('Ctrl Pts',(181.929548894861,6.12347656629904,-107.932368583756));
#20375=CARTESIAN_POINT('Ctrl Pts',(181.931756564295,6.11728427347274,-107.931892853576));
#20376=CARTESIAN_POINT('Ctrl Pts',(181.933762972264,6.11165176399886,-107.931453129964));
#20377=CARTESIAN_POINT('Ctrl Pts',(181.935639441692,6.10638402583803,-107.931041883635));
#20378=CARTESIAN_POINT('Ctrl Pts',(181.937339740164,6.10160632696724,-107.930662212485));
#20379=CARTESIAN_POINT('Ctrl Pts',(181.938858590785,6.09733604159958,-107.930318939573));
#20380=CARTESIAN_POINT('Ctrl Pts',(181.940271356321,6.09336401702112,-107.929999642775));
#20381=CARTESIAN_POINT('Ctrl Pts',(181.941527100859,6.08983111529414,-107.929711865469));
#20382=CARTESIAN_POINT('Ctrl Pts',(181.942636283578,6.0867095443179,-107.929455527493));
#20383=CARTESIAN_POINT('Ctrl Pts',(181.943711826412,6.08368264601373,-107.929206963871));
#20384=CARTESIAN_POINT('Ctrl Pts',(181.944649464688,6.08104279063139,-107.928987991027));
#20385=CARTESIAN_POINT('Ctrl Pts',(181.945474151593,6.07872068925136,-107.928794234602));
#20386=CARTESIAN_POINT('Ctrl Pts',(181.946277169405,6.07645960233774,-107.928605569231));
#20387=CARTESIAN_POINT('Ctrl Pts',(181.946973009188,6.07450002927844,-107.92844082974));
#20388=CARTESIAN_POINT('Ctrl Pts',(181.947600884013,6.07273187234834,-107.928291502419));
#20389=CARTESIAN_POINT('Ctrl Pts',(181.948209135317,6.07101897717428,-107.928146842155));
#20390=CARTESIAN_POINT('Ctrl Pts',(181.948753555853,6.06948585391396,-107.928016653354));
#20391=CARTESIAN_POINT('Ctrl Pts',(181.949286107487,6.06798592939739,-107.927888777429));
#20392=CARTESIAN_POINT('Ctrl Pts',(181.949374353366,6.06773738606642,-107.92786758789));
#20393=CARTESIAN_POINT('Ctrl Pts',(181.94946231164,6.06748964522795,-107.927846451563));
#20394=CARTESIAN_POINT('Ctrl Pts',(181.949550265183,6.06724190764557,-107.927825300627));
#20395=CARTESIAN_POINT('Ctrl Pts',(181.574975446846,5.93046313286183,-107.949597038478));
#20396=CARTESIAN_POINT('Ctrl Pts',(181.699833719625,5.97605605778975,-107.942339792527));
#20397=CARTESIAN_POINT('Ctrl Pts',(181.824691992404,6.02164898271766,-107.935082546577));
#20398=CARTESIAN_POINT('Ctrl Pts',(181.949550265183,6.06724190764558,-107.927825300627));
#20399=CARTESIAN_POINT('',(181.656041870516,6.29154759474223,-107.95));
#20400=CARTESIAN_POINT('Ctrl Pts',(181.5749753816,0.000402959451920593,
-102.019536688494));
#20401=CARTESIAN_POINT('Ctrl Pts',(181.574443965076,0.000386092815958592,
-102.018081442042));
#20402=CARTESIAN_POINT('Ctrl Pts',(181.57276933122,0.000327472074650577,
-102.01349565333));
#20403=CARTESIAN_POINT('Ctrl Pts',(181.565835797325,0.000156658918309325,
-101.994508210116));
#20404=CARTESIAN_POINT('Ctrl Pts',(181.560224999407,5.96987181011011E-5,
-101.97914239978));
#20405=CARTESIAN_POINT('Ctrl Pts',(181.554178400524,7.80232307688747E-6,
-101.962582937518));
#20406=CARTESIAN_POINT('Ctrl Pts',(181.550613625885,-3.04359490813502E-7,
-101.952820381474));
#20407=CARTESIAN_POINT('Ctrl Pts',(181.549938040358,7.48801562377757E-30,
-101.950970255468));
#20408=CARTESIAN_POINT('Ctrl Pts',(181.549583741031,7.48801562377757E-30,
-101.95));
#20409=CARTESIAN_POINT('Ctrl Pts',(181.69983365453,0.00766020089857859,
-101.973943762289));
#20410=CARTESIAN_POINT('Ctrl Pts',(181.698186781027,0.00757264579072308,
-101.969370599695));
#20411=CARTESIAN_POINT('Ctrl Pts',(181.691729730125,0.00689126727407931,
-101.95154639469));
#20412=CARTESIAN_POINT('Ctrl Pts',(181.672686601652,0.00496913839755225,
-101.899121401405));
#20413=CARTESIAN_POINT('Ctrl Pts',(181.652733689967,0.00276020645176135,
-101.844187926299));
#20414=CARTESIAN_POINT('Ctrl Pts',(181.635298291474,0.00110271920042685,
-101.79621853881));
#20415=CARTESIAN_POINT('Ctrl Pts',(181.624637545854,0.000211744708212053,
-101.766881865813));
#20416=CARTESIAN_POINT('Ctrl Pts',(181.621664005803,1.85037170770867E-16,
-101.758689606456));
#20417=CARTESIAN_POINT('Ctrl Pts',(181.620555827354,1.85037170770867E-16,
-101.755634936838));
#20418=CARTESIAN_POINT('Ctrl Pts',(181.82469192746,0.0149174423452366,-101.928350836085));
#20419=CARTESIAN_POINT('Ctrl Pts',(181.821936829738,0.0145269932961417,
-101.920642603346));
#20420=CARTESIAN_POINT('Ctrl Pts',(181.814360476815,0.012485571334149,-101.89983249948));
#20421=CARTESIAN_POINT('Ctrl Pts',(181.7748633369,0.00738273680960432,-101.792464040696));
#20422=CARTESIAN_POINT('Ctrl Pts',(181.74795211748,0.00313538503982533,
-101.718085227754));
#20423=CARTESIAN_POINT('Ctrl Pts',(181.714872511107,0.00102928842360235,
-101.62668976236));
#20424=CARTESIAN_POINT('Ctrl Pts',(181.695960435895,0.000407368516516136,
-101.573825817795));
#20425=CARTESIAN_POINT('Ctrl Pts',(181.693389971248,3.70074341541726E-16,
-101.566408957444));
#20426=CARTESIAN_POINT('Ctrl Pts',(181.691527913677,3.70074341541726E-16,
-101.561269873677));
#20427=CARTESIAN_POINT('Ctrl Pts',(181.949550200389,0.0221746837918946,
-101.88275790988));
#20428=CARTESIAN_POINT('Ctrl Pts',(181.945710620478,0.0212513476946085,
-101.871943016518));
#20429=CARTESIAN_POINT('Ctrl Pts',(181.933702897428,0.0180564544770989,
-101.837905214242));
#20430=CARTESIAN_POINT('Ctrl Pts',(181.883188323836,0.00868662858135192,
-101.69710180877));
#20431=CARTESIAN_POINT('Ctrl Pts',(181.841629490353,0.00330219114123234,
-101.583147980247));
#20432=CARTESIAN_POINT('Ctrl Pts',(181.796617064414,0.000429725518060977,
-101.460332943123));
#20433=CARTESIAN_POINT('Ctrl Pts',(181.770116550723,-1.66216652364724E-5,
-101.387888909435));
#20434=CARTESIAN_POINT('Ctrl Pts',(181.765115936694,5.55111512312586E-16,
-101.374128308432));
#20435=CARTESIAN_POINT('Ctrl Pts',(181.7625,5.55111512312586E-16,-101.366904810515));
#20436=CARTESIAN_POINT('Ctrl Pts',(181.949550200389,0.0221746837918946,
-101.88275790988));
#20437=CARTESIAN_POINT('Ctrl Pts',(181.82469192746,0.0149174423452366,-101.928350836085));
#20438=CARTESIAN_POINT('Ctrl Pts',(181.69983365453,0.00766020089857859,
-101.973943762289));
#20439=CARTESIAN_POINT('Ctrl Pts',(181.5749753816,0.000402959451920593,
-102.019536688494));
#20440=CARTESIAN_POINT('Ctrl Pts',(181.949550200389,0.022174683791894,-101.88275790988));
#20441=CARTESIAN_POINT('Ctrl Pts',(182.135056739364,0.0667850025429474,
-102.405271696106));
#20442=CARTESIAN_POINT('Ctrl Pts',(182.334918859392,0.201307103612158,-103.02537106626));
#20443=CARTESIAN_POINT('Ctrl Pts',(182.51023714977,0.488966122920897,-103.849303636982));
#20444=CARTESIAN_POINT('Ctrl Pts',(182.562500000222,0.638342237723529,-104.202816978021));
#20445=CARTESIAN_POINT('Ctrl Pts',(182.5625,0.800000001098851,-104.521316839394));
#20446=CARTESIAN_POINT('Ctrl Pts',(181.82469192746,0.0149174423452362,-101.928350836085));
#20447=CARTESIAN_POINT('Ctrl Pts',(182.011623315591,0.0465940030836249,
-102.450915459268));
#20448=CARTESIAN_POINT('Ctrl Pts',(182.220049796037,0.16673434696279,-103.0697264493));
#20449=CARTESIAN_POINT('Ctrl Pts',(182.415137827969,0.439989493930775,-103.889969301735));
#20450=CARTESIAN_POINT('Ctrl Pts',(182.477698497991,0.584280425728914,-104.2414573299));
#20451=CARTESIAN_POINT('Ctrl Pts',(182.489526917752,0.743827074166968,-104.557333471973));
#20452=CARTESIAN_POINT('Ctrl Pts',(181.69983365453,0.0076602008985784,-101.973943762289));
#20453=CARTESIAN_POINT('Ctrl Pts',(181.889202893271,0.0266495749489156,
-102.496369000122));
#20454=CARTESIAN_POINT('Ctrl Pts',(182.105417475816,0.132287381924616,-103.114033376099));
#20455=CARTESIAN_POINT('Ctrl Pts',(182.319938028905,0.390946554928068,-103.930656470914));
#20456=CARTESIAN_POINT('Ctrl Pts',(182.393341358782,0.530467074309935,-104.280008116939));
#20457=CARTESIAN_POINT('Ctrl Pts',(182.416553835504,0.687654147235085,-104.593350104552));
#20458=CARTESIAN_POINT('Ctrl Pts',(181.5749753816,0.000402959451920593,
-102.019536688494));
#20459=CARTESIAN_POINT('Ctrl Pts',(181.765769469498,0.0064585754895931,
-102.542012763284));
#20460=CARTESIAN_POINT('Ctrl Pts',(181.990548412461,0.0977146252752476,
-103.158388759139));
#20461=CARTESIAN_POINT('Ctrl Pts',(182.224838707103,0.341969925937946,-103.971322135667));
#20462=CARTESIAN_POINT('Ctrl Pts',(182.308539856551,0.47640526231532,-104.318648468817));
#20463=CARTESIAN_POINT('Ctrl Pts',(182.343580753256,0.631481220303202,-104.629366737131));
#20464=CARTESIAN_POINT('',(182.343580753256,0.631481220303021,-104.62936673713));
#20465=CARTESIAN_POINT('Origin',(182.4625,6.00000000000001,-101.95));
#20466=CARTESIAN_POINT('',(182.5625,3.10645162089483,-106.976666666667));
#20467=CARTESIAN_POINT('',(182.3625,3.00667409058086,-107.15));
#20468=CARTESIAN_POINT('',(182.5625,0.97333333333333,-104.843548379105));
#20469=CARTESIAN_POINT('Origin',(182.5625,6.00000000000001,-101.95));
#20470=CARTESIAN_POINT('',(182.5625,0.97333333333333,-104.843548379105));
#20471=CARTESIAN_POINT('Ctrl Pts',(182.5625,0.800000001098678,-104.521316839393));
#20472=CARTESIAN_POINT('Ctrl Pts',(182.5625,0.857236572714195,-104.634084947445));
#20473=CARTESIAN_POINT('Ctrl Pts',(182.5625,0.91490965910188,-104.742054884846));
#20474=CARTESIAN_POINT('Ctrl Pts',(182.5625,0.973333333333333,-104.843548379105));
#20475=CARTESIAN_POINT('Ctrl Pts',(182.489526917752,0.743827074166794,-104.557333471972));
#20476=CARTESIAN_POINT('Ctrl Pts',(182.49366244611,0.800286860789329,-104.669183196029));
#20477=CARTESIAN_POINT('Ctrl Pts',(182.495833333333,0.857713879611466,-104.77632510792));
#20478=CARTESIAN_POINT('Ctrl Pts',(182.495833333333,0.915555555555554,-104.876807555876));
#20479=CARTESIAN_POINT('Ctrl Pts',(182.416553835504,0.68765414723491,-104.593350104551));
#20480=CARTESIAN_POINT('Ctrl Pts',(182.42482489222,0.743337148864462,-104.704281444612));
#20481=CARTESIAN_POINT('Ctrl Pts',(182.429166666667,0.800518100121053,-104.810595330995));
#20482=CARTESIAN_POINT('Ctrl Pts',(182.429166666667,0.857777777777776,-104.910066732648));
#20483=CARTESIAN_POINT('Ctrl Pts',(182.343580753256,0.631481220303025,-104.62936673713));
#20484=CARTESIAN_POINT('Ctrl Pts',(182.355987338329,0.686387436939596,-104.739379693196));
#20485=CARTESIAN_POINT('Ctrl Pts',(182.3625,0.743322320630639,-104.844865554069));
#20486=CARTESIAN_POINT('Ctrl Pts',(182.3625,0.799999999999998,-104.943325909419));
#20487=CARTESIAN_POINT('Ctrl Pts',(182.5625,0.973333333333333,-104.843548379105));
#20488=CARTESIAN_POINT('Ctrl Pts',(182.5625,0.91490965910188,-104.742054884846));
#20489=CARTESIAN_POINT('Ctrl Pts',(182.5625,0.857236572714195,-104.634084947445));
#20490=CARTESIAN_POINT('Ctrl Pts',(182.5625,0.800000001098678,-104.521316839393));
#20491=CARTESIAN_POINT('Ctrl Pts',(182.5625,3.42868316199153,-107.149999999604));
#20492=CARTESIAN_POINT('Ctrl Pts',(182.562500000088,3.77824139277388,-107.327421746315));
#20493=CARTESIAN_POINT('Ctrl Pts',(182.504123937514,4.15716103788152,-107.487588700127));
#20494=CARTESIAN_POINT('Ctrl Pts',(182.295726889837,5.0552401086783,-107.780573645068));
#20495=CARTESIAN_POINT('Ctrl Pts',(182.122028319689,5.58142525423399,-107.886348035992));
#20496=CARTESIAN_POINT('Ctrl Pts',(181.949550265183,6.06724190764558,-107.927825300627));
#20497=CARTESIAN_POINT('Ctrl Pts',(182.489526917701,3.39266652940122,-107.206172926527));
#20498=CARTESIAN_POINT('Ctrl Pts',(182.476676711164,3.73937765477566,-107.381196742291));
#20499=CARTESIAN_POINT('Ctrl Pts',(182.407104407393,4.11610767175364,-107.535902098076));
#20500=CARTESIAN_POINT('Ctrl Pts',(182.178885909604,5.010573392444,-107.812220832665));
#20501=CARTESIAN_POINT('Ctrl Pts',(181.998732959996,5.5358352609817,-107.905551823336));
#20502=CARTESIAN_POINT('Ctrl Pts',(181.824691992404,6.02164898271766,-107.935082546577));
#20503=CARTESIAN_POINT('Ctrl Pts',(182.416553835402,3.3566498968109,-107.262345853449));
#20504=CARTESIAN_POINT('Ctrl Pts',(182.39094614805,3.70051482143434,-107.434941903931));
#20505=CARTESIAN_POINT('Ctrl Pts',(182.310082495261,4.07505274004195,-107.584215561193));
#20506=CARTESIAN_POINT('Ctrl Pts',(182.062102077776,4.96591130301164,-107.843861421252));
#20507=CARTESIAN_POINT('Ctrl Pts',(181.875666502886,5.49026758092219,-107.924762872177));
#20508=CARTESIAN_POINT('Ctrl Pts',(181.699833719625,5.97605605778975,-107.942339792527));
#20509=CARTESIAN_POINT('Ctrl Pts',(182.343580753104,3.32063326422059,-107.318518780371));
#20510=CARTESIAN_POINT('Ctrl Pts',(182.305122859126,3.66165108343612,-107.488716899907));
#20511=CARTESIAN_POINT('Ctrl Pts',(182.21306296514,4.03399937391406,-107.632528959141));
#20512=CARTESIAN_POINT('Ctrl Pts',(181.945261097542,4.92124458677734,-107.875508608848));
#20513=CARTESIAN_POINT('Ctrl Pts',(181.752371143193,5.4446775876699,-107.943966659521));
#20514=CARTESIAN_POINT('Ctrl Pts',(181.574975446846,5.93046313286183,-107.949597038478));
#20515=CARTESIAN_POINT('',(182.5625,3.42868316190269,-107.14999999978));
#20516=CARTESIAN_POINT('Ctrl Pts',(181.949550265183,6.06724190764558,-107.927825300627));
#20517=CARTESIAN_POINT('Ctrl Pts',(182.122028319689,5.58142525423399,-107.886348035992));
#20518=CARTESIAN_POINT('Ctrl Pts',(182.295726889837,5.0552401086783,-107.780573645068));
#20519=CARTESIAN_POINT('Ctrl Pts',(182.504123937514,4.15716103788152,-107.487588700127));
#20520=CARTESIAN_POINT('Ctrl Pts',(182.562500000088,3.77824139277388,-107.327421746315));
#20521=CARTESIAN_POINT('Ctrl Pts',(182.5625,3.42868316199153,-107.149999999604));
#20522=CARTESIAN_POINT('',(182.5625,3.42868316190269,-107.14999999978));
#20523=CARTESIAN_POINT('Ctrl Pts',(182.5625,3.10645162089484,-106.976666666667));
#20524=CARTESIAN_POINT('Ctrl Pts',(182.5625,3.21069598181732,-107.036673848678));
#20525=CARTESIAN_POINT('Ctrl Pts',(182.5625,3.3180193133645,-107.093831465749));
#20526=CARTESIAN_POINT('Ctrl Pts',(182.5625,3.42868316199166,-107.149999999604));
#20527=CARTESIAN_POINT('Ctrl Pts',(182.495833333333,3.07319244412351,-107.034444444444));
#20528=CARTESIAN_POINT('Ctrl Pts',(182.495833333333,3.17639835547358,-107.093853853762));
#20529=CARTESIAN_POINT('Ctrl Pts',(182.493585276875,3.28290392767116,-107.150766682816));
#20530=CARTESIAN_POINT('Ctrl Pts',(182.489526917701,3.39266652940134,-107.206172926527));
#20531=CARTESIAN_POINT('Ctrl Pts',(182.429166666667,3.03993326735219,-107.092222222222));
#20532=CARTESIAN_POINT('Ctrl Pts',(182.429166666667,3.14210072912985,-107.151033858845));
#20533=CARTESIAN_POINT('Ctrl Pts',(182.424670553749,3.24778854197781,-107.207701899883));
#20534=CARTESIAN_POINT('Ctrl Pts',(182.416553835402,3.35664989681103,-107.262345853449));
#20535=CARTESIAN_POINT('Ctrl Pts',(182.3625,3.00667409058087,-107.15));
#20536=CARTESIAN_POINT('Ctrl Pts',(182.3625,3.10780310278612,-107.208213863928));
#20537=CARTESIAN_POINT('Ctrl Pts',(182.355755830624,3.21267315628447,-107.26463711695));
#20538=CARTESIAN_POINT('Ctrl Pts',(182.343580753104,3.32063326422071,-107.318518780371));
#20539=CARTESIAN_POINT('Ctrl Pts',(182.5625,3.42868316199166,-107.149999999604));
#20540=CARTESIAN_POINT('Ctrl Pts',(182.5625,3.3180193133645,-107.093831465749));
#20541=CARTESIAN_POINT('Ctrl Pts',(182.5625,3.21069598181732,-107.036673848678));
#20542=CARTESIAN_POINT('Ctrl Pts',(182.5625,3.10645162089484,-106.976666666667));
#20543=CARTESIAN_POINT('Origin',(182.5625,63.5,-31.75));
#20544=CARTESIAN_POINT('',(182.5625,123.993325909419,-107.15));
#20545=CARTESIAN_POINT('',(182.5625,34.75,-107.15));
#20546=CARTESIAN_POINT('',(182.5625,126.2,-104.943325909419));
#20547=CARTESIAN_POINT('Origin',(182.5625,121.,-101.95));
#20548=CARTESIAN_POINT('',(182.5625,126.2,41.4433259094192));
#20549=CARTESIAN_POINT('',(182.5625,126.2,-66.85));
#20550=CARTESIAN_POINT('',(182.5625,123.993325909419,43.65));
#20551=CARTESIAN_POINT('Origin',(182.5625,121.,38.45));
#20552=CARTESIAN_POINT('',(182.5625,92.25,43.65));
#20553=CARTESIAN_POINT('Origin',(181.7625,34.75,-107.15));
#20554=CARTESIAN_POINT('',(181.7625,121.,-107.95));
#20555=CARTESIAN_POINT('',(181.7625,34.75,-107.95));
#20556=CARTESIAN_POINT('Ctrl Pts',(181.7625,121.,-107.95));
#20557=CARTESIAN_POINT('Ctrl Pts',(181.939990843115,121.486078692623,-107.95));
#20558=CARTESIAN_POINT('Ctrl Pts',(182.134486665857,122.014025751789,-107.887608349819));
#20559=CARTESIAN_POINT('Ctrl Pts',(182.444388077595,123.043713064318,-107.61628036626));
#20560=CARTESIAN_POINT('Ctrl Pts',(182.5625,123.544851663295,-107.408159534737));
#20561=CARTESIAN_POINT('Ctrl Pts',(182.5625,123.993325909419,-107.15));
#20562=CARTESIAN_POINT('Origin',(177.8,121.,-101.95));
#20563=CARTESIAN_POINT('',(178.6,121.,-107.95));
#20564=CARTESIAN_POINT('',(177.8,121.,-107.95));
#20565=CARTESIAN_POINT('Ctrl Pts',(177.8,123.993325909419,-107.15));
#20566=CARTESIAN_POINT('Ctrl Pts',(177.8,123.544851663295,-107.408159534737));
#20567=CARTESIAN_POINT('Ctrl Pts',(177.918111922405,123.043713064318,-107.61628036626));
#20568=CARTESIAN_POINT('Ctrl Pts',(178.228013334143,122.014025751789,-107.887608349819));
#20569=CARTESIAN_POINT('Ctrl Pts',(178.422509156885,121.486078692623,-107.95));
#20570=CARTESIAN_POINT('Ctrl Pts',(178.6,121.,-107.95));
#20571=CARTESIAN_POINT('',(178.6,127.,-101.95));
#20572=CARTESIAN_POINT('Ctrl Pts',(178.6,127.,-101.95));
#20573=CARTESIAN_POINT('Ctrl Pts',(178.422509156885,127.,-102.436078692623));
#20574=CARTESIAN_POINT('Ctrl Pts',(178.228013334143,126.937608349819,-102.964025751789));
#20575=CARTESIAN_POINT('Ctrl Pts',(177.918111922405,126.66628036626,-103.993713064318));
#20576=CARTESIAN_POINT('Ctrl Pts',(177.8,126.458159534737,-104.494851663295));
#20577=CARTESIAN_POINT('Ctrl Pts',(177.8,126.2,-104.943325909419));
#20578=CARTESIAN_POINT('',(181.7625,127.,-101.95));
#20579=CARTESIAN_POINT('',(177.8,127.,-101.95));
#20580=CARTESIAN_POINT('Ctrl Pts',(182.5625,126.2,-104.943325909419));
#20581=CARTESIAN_POINT('Ctrl Pts',(182.5625,126.458159534737,-104.494851663295));
#20582=CARTESIAN_POINT('Ctrl Pts',(182.444388077595,126.66628036626,-103.993713064318));
#20583=CARTESIAN_POINT('Ctrl Pts',(182.134486665857,126.937608349819,-102.964025751789));
#20584=CARTESIAN_POINT('Ctrl Pts',(181.939990843115,127.,-102.436078692623));
#20585=CARTESIAN_POINT('Ctrl Pts',(181.7625,127.,-101.95));
#20586=CARTESIAN_POINT('Origin',(177.8,6.,-107.95));
#20587=CARTESIAN_POINT('',(178.6,34.75,-107.95));
#20588=CARTESIAN_POINT('Origin',(178.6,34.75,-107.15));
#20589=CARTESIAN_POINT('Origin',(181.7625,126.2,-66.85));
#20590=CARTESIAN_POINT('',(181.7625,127.,38.45));
#20591=CARTESIAN_POINT('Ctrl Pts',(181.7625,127.,38.45));
#20592=CARTESIAN_POINT('Ctrl Pts',(181.939990843115,127.,38.9360786926232));
#20593=CARTESIAN_POINT('Ctrl Pts',(182.134486665857,126.937608349819,39.4640257517887));
#20594=CARTESIAN_POINT('Ctrl Pts',(182.444388077595,126.66628036626,40.4937130643181));
#20595=CARTESIAN_POINT('Ctrl Pts',(182.5625,126.458159534737,40.9948516632952));
#20596=CARTESIAN_POINT('Ctrl Pts',(182.5625,126.2,41.4433259094192));
#20597=CARTESIAN_POINT('',(181.7625,127.,-66.85));
#20598=CARTESIAN_POINT('Origin',(177.8,121.,38.45));
#20599=CARTESIAN_POINT('',(178.6,127.,38.45));
#20600=CARTESIAN_POINT('',(177.8,127.,38.45));
#20601=CARTESIAN_POINT('Ctrl Pts',(177.8,126.2,41.4433259094192));
#20602=CARTESIAN_POINT('Ctrl Pts',(177.8,126.458159534737,40.9948516632952));
#20603=CARTESIAN_POINT('Ctrl Pts',(177.918111922405,126.66628036626,40.4937130643181));
#20604=CARTESIAN_POINT('Ctrl Pts',(178.228013334143,126.937608349819,39.4640257517887));
#20605=CARTESIAN_POINT('Ctrl Pts',(178.422509156885,127.,38.9360786926232));
#20606=CARTESIAN_POINT('Ctrl Pts',(178.6,127.,38.45));
#20607=CARTESIAN_POINT('',(178.6,121.,44.45));
#20608=CARTESIAN_POINT('Ctrl Pts',(178.6,121.,44.45));
#20609=CARTESIAN_POINT('Ctrl Pts',(178.40913336376,121.52270981072,44.45));
#20610=CARTESIAN_POINT('Ctrl Pts',(178.182728070533,122.14501659934,44.3640989204313));
#20611=CARTESIAN_POINT('Ctrl Pts',(177.910747095178,123.089471451833,44.0921179450766));
#20612=CARTESIAN_POINT('Ctrl Pts',(177.8,123.591791866647,43.8811388949509));
#20613=CARTESIAN_POINT('Ctrl Pts',(177.8,123.993325909419,43.65));
#20614=CARTESIAN_POINT('',(181.7625,121.,44.45));
#20615=CARTESIAN_POINT('',(177.8,121.,44.45));
#20616=CARTESIAN_POINT('Ctrl Pts',(182.5625,123.993325909419,43.65));
#20617=CARTESIAN_POINT('Ctrl Pts',(182.5625,123.544851663295,43.9081595347366));
#20618=CARTESIAN_POINT('Ctrl Pts',(182.444388077595,123.043713064318,44.1162803662604));
#20619=CARTESIAN_POINT('Ctrl Pts',(182.134486665857,122.014025751789,44.387608349819));
#20620=CARTESIAN_POINT('Ctrl Pts',(181.939990843115,121.486078692623,44.45));
#20621=CARTESIAN_POINT('Ctrl Pts',(181.7625,121.,44.45));
#20622=CARTESIAN_POINT('Origin',(177.8,127.,-101.95));
#20623=CARTESIAN_POINT('',(178.6,127.,-66.85));
#20624=CARTESIAN_POINT('Origin',(178.6,126.2,-66.85));
#20625=CARTESIAN_POINT('Origin',(181.7625,92.25,43.65));
#20626=CARTESIAN_POINT('',(181.7625,92.25,44.45));
#20627=CARTESIAN_POINT('Origin',(177.8,121.,44.45));
#20628=CARTESIAN_POINT('',(178.6,92.25,44.45));
#20629=CARTESIAN_POINT('Origin',(178.6,92.25,43.65));
#32280=UNCERTAINTY_MEASURE_WITH_UNIT(LENGTH_MEASURE(0.01),#32310,
'DISTANCE_ACCURACY_VALUE',
'Maximum model space distance between geometric entities at asserted c
onnectivities');
#32293=UNCERTAINTY_MEASURE_WITH_UNIT(LENGTH_MEASURE(0.01),#32310,
'DISTANCE_ACCURACY_VALUE',
'Maximum model space distance between geometric entities at asserted c
onnectivities');
#32296=(
GEOMETRIC_REPRESENTATION_CONTEXT(3)
GLOBAL_UNCERTAINTY_ASSIGNED_CONTEXT((#32280))
GLOBAL_UNIT_ASSIGNED_CONTEXT((#32310,#32312,#32313))
REPRESENTATION_CONTEXT('','3D')
);
#32309=(
GEOMETRIC_REPRESENTATION_CONTEXT(3)
GLOBAL_UNCERTAINTY_ASSIGNED_CONTEXT((#32293))
GLOBAL_UNIT_ASSIGNED_CONTEXT((#32310,#32312,#32313))
REPRESENTATION_CONTEXT('','3D')
);
#32310=(
LENGTH_UNIT()
NAMED_UNIT(*)
SI_UNIT(.MILLI.,.METRE.)
);
#32312=(
NAMED_UNIT(*)
PLANE_ANGLE_UNIT()
SI_UNIT($,.RADIAN.)
);
#32313=(
NAMED_UNIT(*)
SI_UNIT($,.STERADIAN.)
SOLID_ANGLE_UNIT()
);
#32316=SHAPE_DEFINITION_REPRESENTATION(#32331,#32363);
#32331=PRODUCT_DEFINITION_SHAPE('',$,#32379);
#32363=SHAPE_REPRESENTATION('',(#14060),#32296);
#32376=PRODUCT_DEFINITION_CONTEXT('part definition',#32423,'design');
#32379=PRODUCT_DEFINITION('2026-10-25-00-35-15-886',
'02_Outer_End_Plate_6in',#32394,#32376);
#32394=PRODUCT_DEFINITION_FORMATION('',$,#32427);
#32423=APPLICATION_CONTEXT(
'Core Data for Automotive Mechanical Design Process');
#32424=PRODUCT_CONTEXT('part definition',#32423,'mechanical');
#32427=PRODUCT('2026-10-25-00-35-15-886','02_Outer_End_Plate_6in',$,(#32424));
#32510=COLOUR_RGB('Off White',0.89,0.88,0.83);
#32511=FILL_AREA_STYLE_COLOUR('',#32510);
#32512=FILL_AREA_STYLE('',(#32511));
#32513=SURFACE_STYLE_FILL_AREA(#32512);
#32514=SURFACE_SIDE_STYLE('',(#32513));
#32515=SURFACE_STYLE_USAGE(.BOTH.,#32514);
#32516=PRESENTATION_STYLE_ASSIGNMENT((#32515));
ENDSEC;
END-ISO-10303-21;
